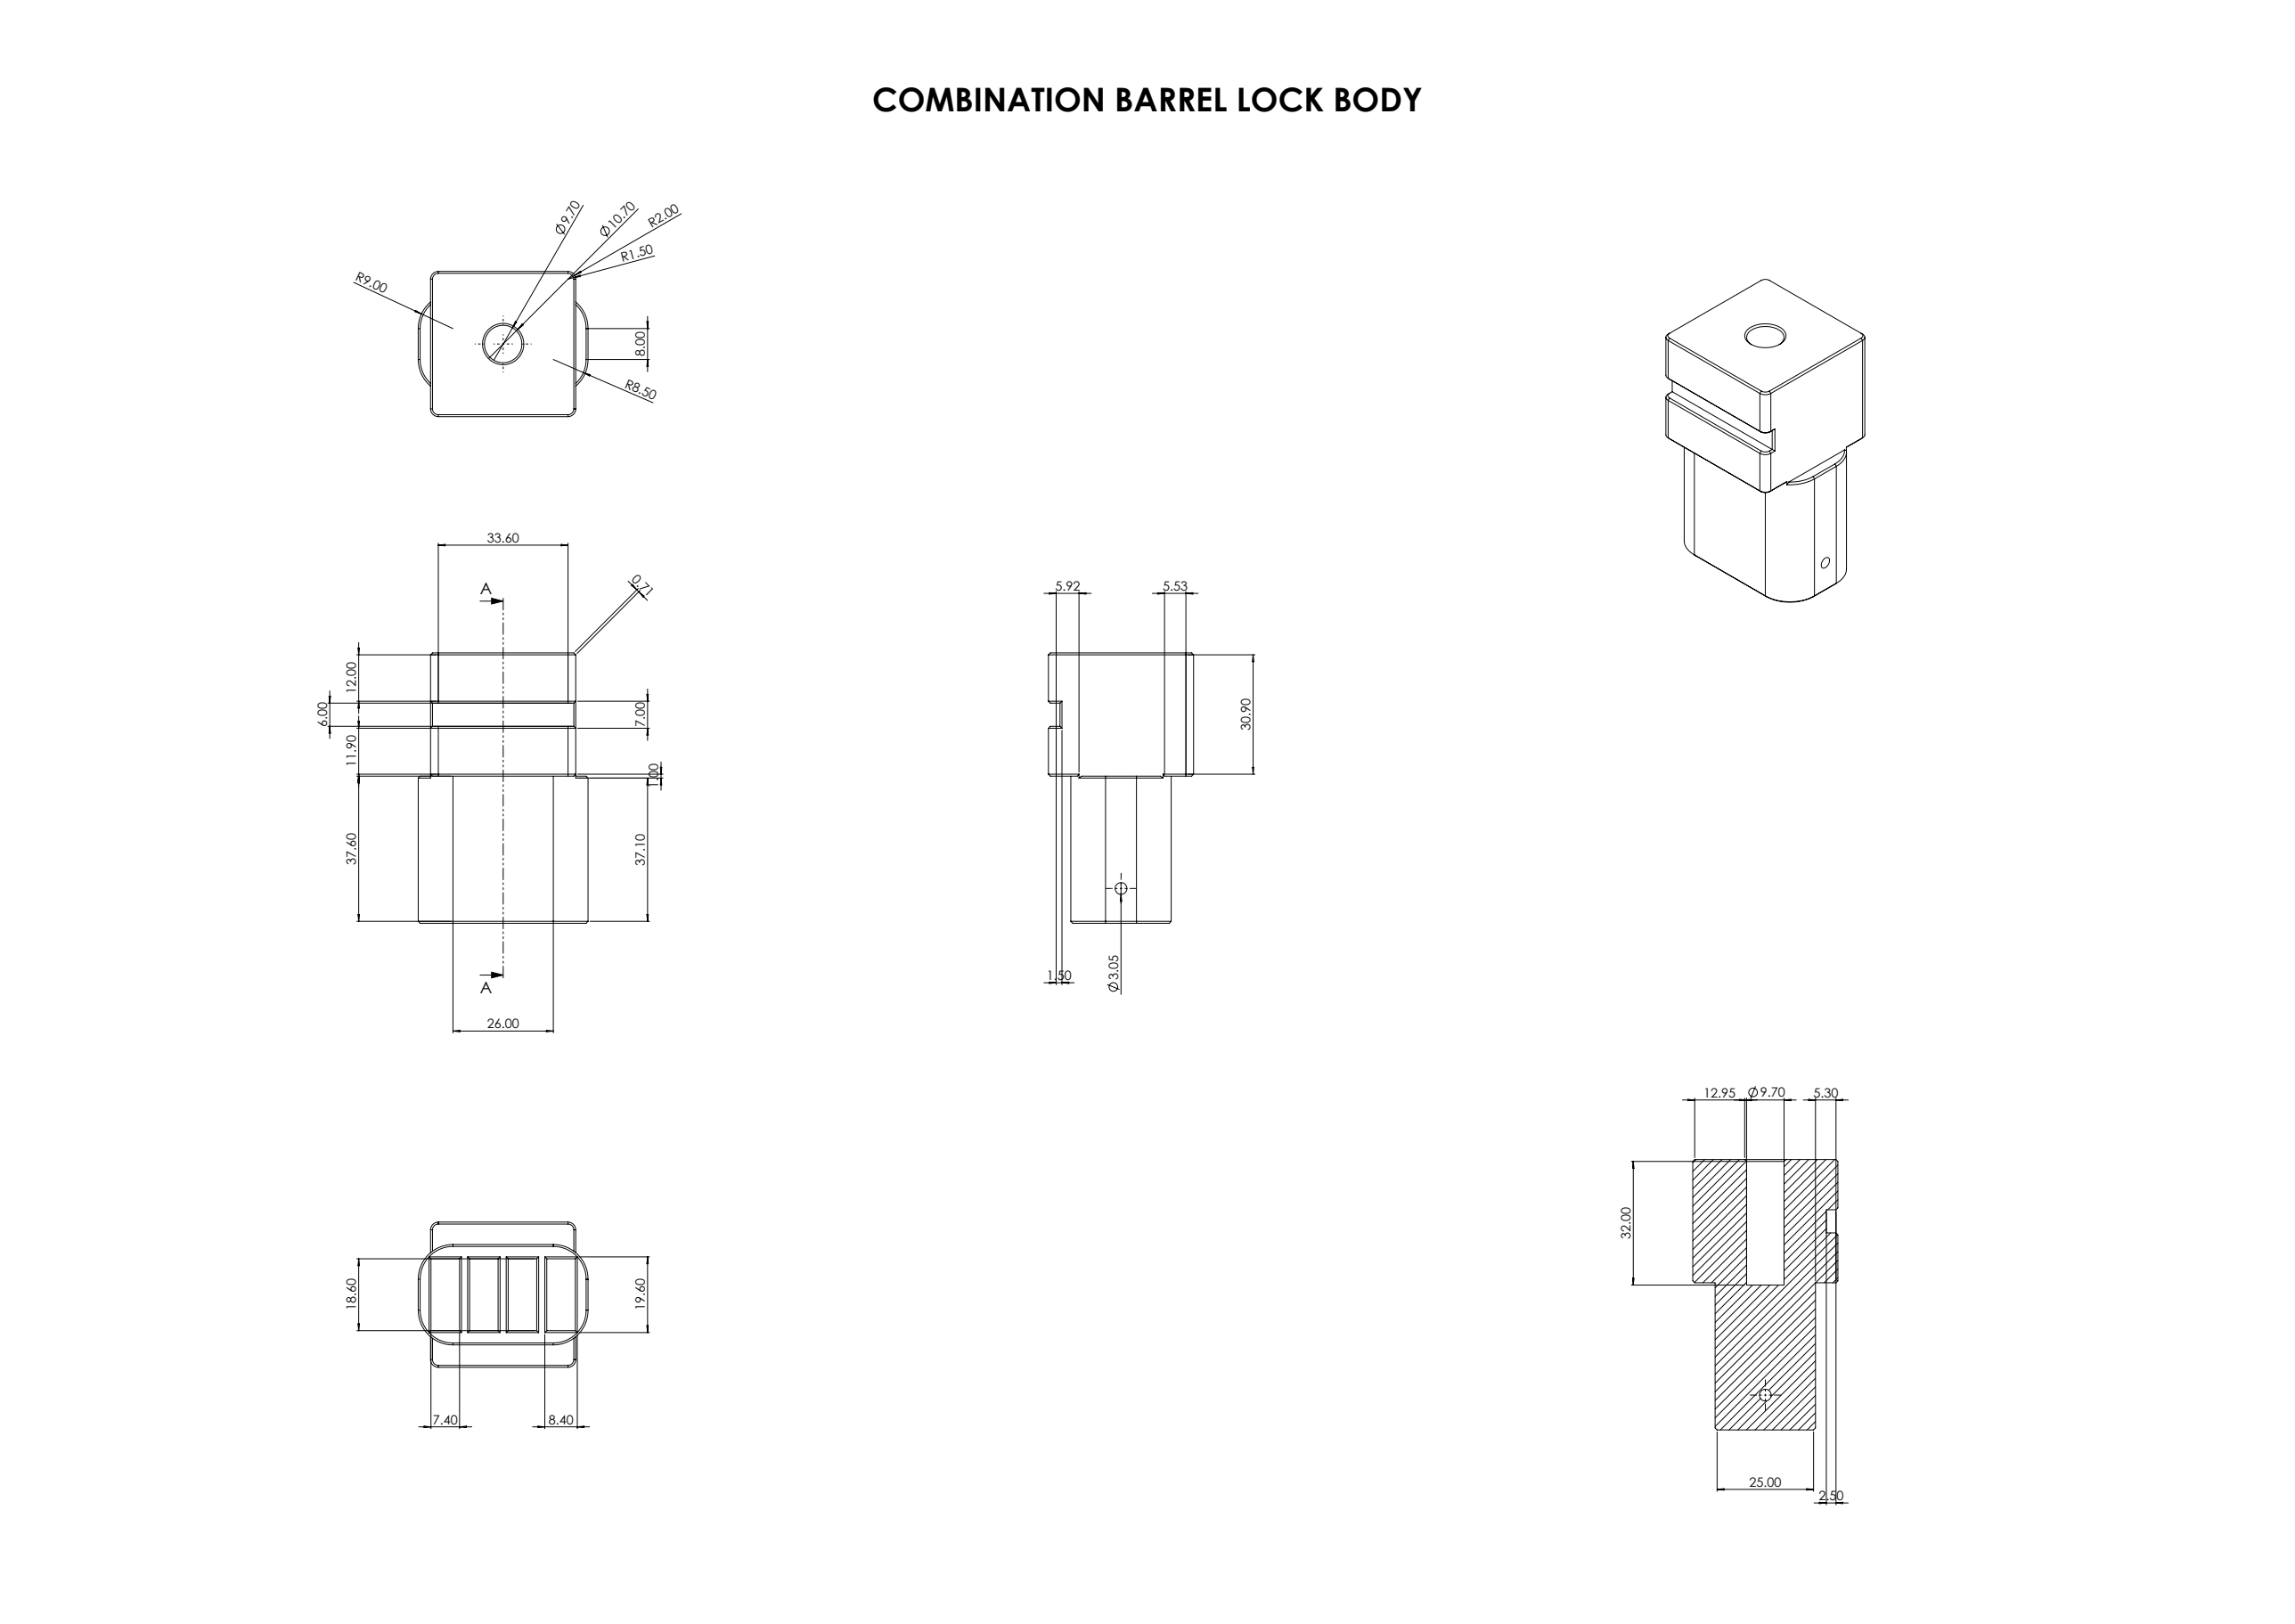
ISO-10303-21;
HEADER;
/* Generated by software containing ST-Developer
 * from STEP Tools, Inc. (www.steptools.com) 
 */

FILE_DESCRIPTION(
/* description */ (''),
/* implementation_level */ '2;1');

FILE_NAME(
/* name */ '08_Combination_Barrel_Lock_Body.step',
/* time_stamp */ '2026-10-25T01:30:15-07:00',
/* author */ (''),
/* organization */ (''),
/* preprocessor_version */ 'ST-DEVELOPER v20.2',
/* originating_system */ 'Autodesk Translation Framework v15.15.0.0',
/* authorisation */ '');

FILE_SCHEMA (('AUTOMOTIVE_DESIGN { 1 0 10303 214 3 1 1 }'));
ENDSEC;

DATA;
#10=MECHANICAL_DESIGN_GEOMETRIC_PRESENTATION_REPRESENTATION('',(#570),#32309);
#79=ELLIPSE('',#14443,12.7279220613578,8.99999999999999);
#80=ELLIPSE('',#14447,12.7279220613579,9.);
#81=ELLIPSE('',#14470,12.7279220613578,9.);
#82=ELLIPSE('',#14474,12.7279220613578,9.);
#83=(
BOUNDED_CURVE()
B_SPLINE_CURVE(2,(#25941,#25942,#25943),.UNSPECIFIED.,.F.,.F.)
B_SPLINE_CURVE_WITH_KNOTS((3,3),(0.,0.083454512499127),.UNSPECIFIED.)
CURVE()
GEOMETRIC_REPRESENTATION_ITEM()
RATIONAL_B_SPLINE_CURVE((1.,1.00072968826169,1.))
REPRESENTATION_ITEM('')
);
#84=(
BOUNDED_CURVE()
B_SPLINE_CURVE(2,(#25958,#25959,#25960),.UNSPECIFIED.,.F.,.F.)
B_SPLINE_CURVE_WITH_KNOTS((3,3),(0.,0.0834545124991277),.UNSPECIFIED.)
CURVE()
GEOMETRIC_REPRESENTATION_ITEM()
RATIONAL_B_SPLINE_CURVE((1.,1.00072968826163,1.))
REPRESENTATION_ITEM('')
);
#85=(
BOUNDED_CURVE()
B_SPLINE_CURVE(2,(#26021,#26022,#26023),.UNSPECIFIED.,.F.,.F.)
B_SPLINE_CURVE_WITH_KNOTS((3,3),(0.,0.0834545124991279),.UNSPECIFIED.)
CURVE()
GEOMETRIC_REPRESENTATION_ITEM()
RATIONAL_B_SPLINE_CURVE((1.,1.00072968826024,1.))
REPRESENTATION_ITEM('')
);
#86=(
BOUNDED_CURVE()
B_SPLINE_CURVE(2,(#26038,#26039,#26040),.UNSPECIFIED.,.F.,.F.)
B_SPLINE_CURVE_WITH_KNOTS((3,3),(0.,0.083454512499128),.UNSPECIFIED.)
CURVE()
GEOMETRIC_REPRESENTATION_ITEM()
RATIONAL_B_SPLINE_CURVE((1.,1.0007296882565,1.))
REPRESENTATION_ITEM('')
);
#542=SHAPE_REPRESENTATION_RELATIONSHIP('SRR','None',#32369,#556);
#556=ADVANCED_BREP_SHAPE_REPRESENTATION('',(#584),#32302);
#570=STYLED_ITEM('',(#32481),#584);
#584=MANIFOLD_SOLID_BREP('Body1',#13811);
#627=FACE_BOUND('',#2435,.T.);
#628=FACE_BOUND('',#2439,.T.);
#629=FACE_BOUND('',#2446,.T.);
#630=FACE_BOUND('',#2488,.T.);
#631=FACE_BOUND('',#2489,.T.);
#632=FACE_BOUND('',#2490,.T.);
#633=FACE_BOUND('',#2491,.T.);
#634=FACE_BOUND('',#2510,.T.);
#635=FACE_BOUND('',#2517,.T.);
#636=FACE_BOUND('',#2524,.T.);
#637=FACE_BOUND('',#2531,.T.);
#638=FACE_BOUND('',#2539,.T.);
#639=FACE_BOUND('',#2543,.T.);
#640=FACE_BOUND('',#2547,.T.);
#641=FACE_BOUND('',#2551,.T.);
#726=CYLINDRICAL_SURFACE('',#14440,8.99999999999999);
#727=CYLINDRICAL_SURFACE('',#14446,9.);
#728=CYLINDRICAL_SURFACE('',#14458,4.85);
#729=CYLINDRICAL_SURFACE('',#14467,9.);
#730=CYLINDRICAL_SURFACE('',#14473,9.);
#731=CYLINDRICAL_SURFACE('',#14487,2.);
#732=CYLINDRICAL_SURFACE('',#14490,2.);
#733=CYLINDRICAL_SURFACE('',#14502,2.);
#734=CYLINDRICAL_SURFACE('',#14505,2.);
#735=CYLINDRICAL_SURFACE('',#14517,2.);
#736=CYLINDRICAL_SURFACE('',#14581,1.525);
#737=CYLINDRICAL_SURFACE('',#14583,1.525);
#738=CYLINDRICAL_SURFACE('',#14585,1.525);
#739=CYLINDRICAL_SURFACE('',#14587,1.525);
#740=CYLINDRICAL_SURFACE('',#14589,1.525);
#741=CYLINDRICAL_SURFACE('',#14603,2.);
#951=CIRCLE('',#14434,9.);
#952=CIRCLE('',#14435,8.5);
#953=CIRCLE('',#14438,8.49999999999999);
#954=CIRCLE('',#14439,8.99999999999999);
#955=CIRCLE('',#14441,8.99999999999999);
#956=CIRCLE('',#14442,8.99999999999999);
#957=CIRCLE('',#14445,1.525);
#958=CIRCLE('',#14448,9.);
#959=CIRCLE('',#14449,9.);
#960=CIRCLE('',#14451,5.35);
#961=CIRCLE('',#14452,4.85);
#962=CIRCLE('',#14454,1.5);
#963=CIRCLE('',#14455,1.5);
#964=CIRCLE('',#14456,1.5);
#965=CIRCLE('',#14457,1.5);
#966=CIRCLE('',#14459,4.85);
#967=CIRCLE('',#14461,9.);
#968=CIRCLE('',#14462,8.5);
#969=CIRCLE('',#14465,8.5);
#970=CIRCLE('',#14466,9.);
#971=CIRCLE('',#14468,9.);
#972=CIRCLE('',#14469,9.);
#973=CIRCLE('',#14472,1.525);
#974=CIRCLE('',#14475,9.);
#975=CIRCLE('',#14476,9.);
#976=CIRCLE('',#14479,1.5);
#977=CIRCLE('',#14480,2.);
#978=CIRCLE('',#14483,1.5);
#979=CIRCLE('',#14484,2.);
#980=CIRCLE('',#14488,2.);
#981=CIRCLE('',#14491,2.);
#982=CIRCLE('',#14495,1.5);
#983=CIRCLE('',#14496,2.);
#984=CIRCLE('',#14499,1.5);
#985=CIRCLE('',#14500,2.);
#986=CIRCLE('',#14503,2.);
#987=CIRCLE('',#14506,2.);
#988=CIRCLE('',#14508,2.);
#989=CIRCLE('',#14515,2.);
#990=CIRCLE('',#14518,2.);
#991=CIRCLE('',#14523,8.49999999999999);
#992=CIRCLE('',#14526,8.5);
#993=CIRCLE('',#14529,8.5);
#994=CIRCLE('',#14532,8.5);
#995=CIRCLE('',#14538,2.);
#996=CIRCLE('',#14539,1.5);
#997=CIRCLE('',#14542,1.5);
#998=CIRCLE('',#14547,1.5);
#999=CIRCLE('',#14550,1.5);
#1000=CIRCLE('',#14559,1.525);
#1001=CIRCLE('',#14566,1.525);
#1002=CIRCLE('',#14573,1.525);
#1003=CIRCLE('',#14580,1.525);
#1004=CIRCLE('',#14582,1.525);
#1005=CIRCLE('',#14584,1.525);
#1006=CIRCLE('',#14586,1.525);
#1007=CIRCLE('',#14588,1.525);
#1181=CONICAL_SURFACE('',#14433,8.75,0.785398163397444);
#1182=CONICAL_SURFACE('',#14437,8.75,0.785398163397449);
#1183=CONICAL_SURFACE('',#14450,5.1,0.785398163397447);
#1184=CONICAL_SURFACE('',#14460,8.75,0.785398163397449);
#1185=CONICAL_SURFACE('',#14464,8.75,0.785398163397451);
#1186=CONICAL_SURFACE('',#14478,1.75,0.785398163397449);
#1187=CONICAL_SURFACE('',#14482,1.75,0.785398163397449);
#1188=CONICAL_SURFACE('',#14494,1.75,0.785398163397449);
#1189=CONICAL_SURFACE('',#14498,1.75,0.785398163397449);
#1190=CONICAL_SURFACE('',#14507,1.75,0.785398163397447);
#1191=CONICAL_SURFACE('',#14510,1.75,0.785398163397447);
#1192=CONICAL_SURFACE('',#14512,1.75,0.785398163397447);
#1193=CONICAL_SURFACE('',#14514,1.75,0.785398163397447);
#1194=CONICAL_SURFACE('',#14522,8.75,0.785398163397449);
#1195=CONICAL_SURFACE('',#14525,8.75,0.785398163397449);
#1196=CONICAL_SURFACE('',#14528,8.75,0.785398163397449);
#1197=CONICAL_SURFACE('',#14531,8.75,0.785398163397449);
#1198=CONICAL_SURFACE('',#14537,1.75,0.785398163397447);
#1199=CONICAL_SURFACE('',#14541,1.75,0.785398163397447);
#1200=CONICAL_SURFACE('',#14546,1.75,0.785398163397447);
#1201=CONICAL_SURFACE('',#14549,1.75,0.785398163397447);
#1595=FACE_OUTER_BOUND('',#2430,.T.);
#1596=FACE_OUTER_BOUND('',#2431,.T.);
#1597=FACE_OUTER_BOUND('',#2432,.T.);
#1598=FACE_OUTER_BOUND('',#2433,.T.);
#1599=FACE_OUTER_BOUND('',#2434,.T.);
#1600=FACE_OUTER_BOUND('',#2436,.T.);
#1601=FACE_OUTER_BOUND('',#2437,.T.);
#1602=FACE_OUTER_BOUND('',#2438,.T.);
#1603=FACE_OUTER_BOUND('',#2440,.T.);
#1604=FACE_OUTER_BOUND('',#2441,.T.);
#1605=FACE_OUTER_BOUND('',#2442,.T.);
#1606=FACE_OUTER_BOUND('',#2443,.T.);
#1607=FACE_OUTER_BOUND('',#2444,.T.);
#1608=FACE_OUTER_BOUND('',#2445,.T.);
#1609=FACE_OUTER_BOUND('',#2447,.T.);
#1610=FACE_OUTER_BOUND('',#2448,.T.);
#1611=FACE_OUTER_BOUND('',#2449,.T.);
#1612=FACE_OUTER_BOUND('',#2450,.T.);
#1613=FACE_OUTER_BOUND('',#2451,.T.);
#1614=FACE_OUTER_BOUND('',#2452,.T.);
#1615=FACE_OUTER_BOUND('',#2453,.T.);
#1616=FACE_OUTER_BOUND('',#2454,.T.);
#1617=FACE_OUTER_BOUND('',#2455,.T.);
#1618=FACE_OUTER_BOUND('',#2456,.T.);
#1619=FACE_OUTER_BOUND('',#2457,.T.);
#1620=FACE_OUTER_BOUND('',#2458,.T.);
#1621=FACE_OUTER_BOUND('',#2459,.T.);
#1622=FACE_OUTER_BOUND('',#2460,.T.);
#1623=FACE_OUTER_BOUND('',#2461,.T.);
#1624=FACE_OUTER_BOUND('',#2462,.T.);
#1625=FACE_OUTER_BOUND('',#2463,.T.);
#1626=FACE_OUTER_BOUND('',#2464,.T.);
#1627=FACE_OUTER_BOUND('',#2465,.T.);
#1628=FACE_OUTER_BOUND('',#2466,.T.);
#1629=FACE_OUTER_BOUND('',#2467,.T.);
#1630=FACE_OUTER_BOUND('',#2468,.T.);
#1631=FACE_OUTER_BOUND('',#2469,.T.);
#1632=FACE_OUTER_BOUND('',#2470,.T.);
#1633=FACE_OUTER_BOUND('',#2471,.T.);
#1634=FACE_OUTER_BOUND('',#2472,.T.);
#1635=FACE_OUTER_BOUND('',#2473,.T.);
#1636=FACE_OUTER_BOUND('',#2474,.T.);
#1637=FACE_OUTER_BOUND('',#2475,.T.);
#1638=FACE_OUTER_BOUND('',#2476,.T.);
#1639=FACE_OUTER_BOUND('',#2477,.T.);
#1640=FACE_OUTER_BOUND('',#2478,.T.);
#1641=FACE_OUTER_BOUND('',#2479,.T.);
#1642=FACE_OUTER_BOUND('',#2480,.T.);
#1643=FACE_OUTER_BOUND('',#2481,.T.);
#1644=FACE_OUTER_BOUND('',#2482,.T.);
#1645=FACE_OUTER_BOUND('',#2483,.T.);
#1646=FACE_OUTER_BOUND('',#2484,.T.);
#1647=FACE_OUTER_BOUND('',#2485,.T.);
#1648=FACE_OUTER_BOUND('',#2486,.T.);
#1649=FACE_OUTER_BOUND('',#2487,.T.);
#1650=FACE_OUTER_BOUND('',#2492,.T.);
#1651=FACE_OUTER_BOUND('',#2493,.T.);
#1652=FACE_OUTER_BOUND('',#2494,.T.);
#1653=FACE_OUTER_BOUND('',#2495,.T.);
#1654=FACE_OUTER_BOUND('',#2496,.T.);
#1655=FACE_OUTER_BOUND('',#2497,.T.);
#1656=FACE_OUTER_BOUND('',#2498,.T.);
#1657=FACE_OUTER_BOUND('',#2499,.T.);
#1658=FACE_OUTER_BOUND('',#2500,.T.);
#1659=FACE_OUTER_BOUND('',#2501,.T.);
#1660=FACE_OUTER_BOUND('',#2502,.T.);
#1661=FACE_OUTER_BOUND('',#2503,.T.);
#1662=FACE_OUTER_BOUND('',#2504,.T.);
#1663=FACE_OUTER_BOUND('',#2505,.T.);
#1664=FACE_OUTER_BOUND('',#2506,.T.);
#1665=FACE_OUTER_BOUND('',#2507,.T.);
#1666=FACE_OUTER_BOUND('',#2508,.T.);
#1667=FACE_OUTER_BOUND('',#2509,.T.);
#1668=FACE_OUTER_BOUND('',#2511,.T.);
#1669=FACE_OUTER_BOUND('',#2512,.T.);
#1670=FACE_OUTER_BOUND('',#2513,.T.);
#1671=FACE_OUTER_BOUND('',#2514,.T.);
#1672=FACE_OUTER_BOUND('',#2515,.T.);
#1673=FACE_OUTER_BOUND('',#2516,.T.);
#1674=FACE_OUTER_BOUND('',#2518,.T.);
#1675=FACE_OUTER_BOUND('',#2519,.T.);
#1676=FACE_OUTER_BOUND('',#2520,.T.);
#1677=FACE_OUTER_BOUND('',#2521,.T.);
#1678=FACE_OUTER_BOUND('',#2522,.T.);
#1679=FACE_OUTER_BOUND('',#2523,.T.);
#1680=FACE_OUTER_BOUND('',#2525,.T.);
#1681=FACE_OUTER_BOUND('',#2526,.T.);
#1682=FACE_OUTER_BOUND('',#2527,.T.);
#1683=FACE_OUTER_BOUND('',#2528,.T.);
#1684=FACE_OUTER_BOUND('',#2529,.T.);
#1685=FACE_OUTER_BOUND('',#2530,.T.);
#1686=FACE_OUTER_BOUND('',#2532,.T.);
#1687=FACE_OUTER_BOUND('',#2533,.T.);
#1688=FACE_OUTER_BOUND('',#2534,.T.);
#1689=FACE_OUTER_BOUND('',#2535,.T.);
#1690=FACE_OUTER_BOUND('',#2536,.T.);
#1691=FACE_OUTER_BOUND('',#2537,.T.);
#1692=FACE_OUTER_BOUND('',#2538,.T.);
#1693=FACE_OUTER_BOUND('',#2540,.T.);
#1694=FACE_OUTER_BOUND('',#2541,.T.);
#1695=FACE_OUTER_BOUND('',#2542,.T.);
#1696=FACE_OUTER_BOUND('',#2544,.T.);
#1697=FACE_OUTER_BOUND('',#2545,.T.);
#1698=FACE_OUTER_BOUND('',#2546,.T.);
#1699=FACE_OUTER_BOUND('',#2548,.T.);
#1700=FACE_OUTER_BOUND('',#2549,.T.);
#1701=FACE_OUTER_BOUND('',#2550,.T.);
#1702=FACE_OUTER_BOUND('',#2552,.T.);
#1703=FACE_OUTER_BOUND('',#2553,.T.);
#1704=FACE_OUTER_BOUND('',#2554,.T.);
#1705=FACE_OUTER_BOUND('',#2555,.T.);
#1706=FACE_OUTER_BOUND('',#2556,.T.);
#1707=FACE_OUTER_BOUND('',#2557,.T.);
#1708=FACE_OUTER_BOUND('',#2558,.T.);
#1709=FACE_OUTER_BOUND('',#2559,.T.);
#1710=FACE_OUTER_BOUND('',#2560,.T.);
#2430=EDGE_LOOP('',(#10369,#10370,#10371,#10372));
#2431=EDGE_LOOP('',(#10373,#10374,#10375,#10376));
#2432=EDGE_LOOP('',(#10377,#10378,#10379,#10380));
#2433=EDGE_LOOP('',(#10381,#10382,#10383,#10384,#10385,#10386,#10387));
#2434=EDGE_LOOP('',(#10388,#10389,#10390,#10391));
#2435=EDGE_LOOP('',(#10392));
#2436=EDGE_LOOP('',(#10393,#10394,#10395,#10396,#10397,#10398,#10399));
#2437=EDGE_LOOP('',(#10400,#10401,#10402,#10403));
#2438=EDGE_LOOP('',(#10404,#10405,#10406,#10407,#10408,#10409,#10410,#10411));
#2439=EDGE_LOOP('',(#10412));
#2440=EDGE_LOOP('',(#10413,#10414,#10415,#10416));
#2441=EDGE_LOOP('',(#10417,#10418,#10419,#10420));
#2442=EDGE_LOOP('',(#10421,#10422,#10423,#10424));
#2443=EDGE_LOOP('',(#10425,#10426,#10427,#10428));
#2444=EDGE_LOOP('',(#10429,#10430,#10431,#10432,#10433,#10434,#10435));
#2445=EDGE_LOOP('',(#10436,#10437,#10438,#10439));
#2446=EDGE_LOOP('',(#10440));
#2447=EDGE_LOOP('',(#10441,#10442,#10443,#10444,#10445,#10446,#10447));
#2448=EDGE_LOOP('',(#10448,#10449,#10450,#10451));
#2449=EDGE_LOOP('',(#10452,#10453,#10454,#10455));
#2450=EDGE_LOOP('',(#10456,#10457,#10458,#10459));
#2451=EDGE_LOOP('',(#10460,#10461,#10462,#10463));
#2452=EDGE_LOOP('',(#10464,#10465,#10466,#10467));
#2453=EDGE_LOOP('',(#10468,#10469,#10470,#10471,#10472,#10473,#10474,#10475,
#10476,#10477,#10478,#10479,#10480,#10481));
#2454=EDGE_LOOP('',(#10482,#10483,#10484,#10485));
#2455=EDGE_LOOP('',(#10486,#10487,#10488,#10489));
#2456=EDGE_LOOP('',(#10490,#10491,#10492,#10493));
#2457=EDGE_LOOP('',(#10494,#10495,#10496,#10497,#10498,#10499,#10500,#10501,
#10502,#10503,#10504,#10505,#10506,#10507));
#2458=EDGE_LOOP('',(#10508,#10509,#10510,#10511));
#2459=EDGE_LOOP('',(#10512,#10513,#10514,#10515));
#2460=EDGE_LOOP('',(#10516,#10517,#10518,#10519));
#2461=EDGE_LOOP('',(#10520,#10521,#10522,#10523));
#2462=EDGE_LOOP('',(#10524,#10525,#10526,#10527));
#2463=EDGE_LOOP('',(#10528,#10529,#10530,#10531));
#2464=EDGE_LOOP('',(#10532,#10533,#10534,#10535));
#2465=EDGE_LOOP('',(#10536,#10537,#10538,#10539));
#2466=EDGE_LOOP('',(#10540,#10541,#10542,#10543));
#2467=EDGE_LOOP('',(#10544,#10545,#10546,#10547));
#2468=EDGE_LOOP('',(#10548,#10549,#10550,#10551));
#2469=EDGE_LOOP('',(#10552,#10553,#10554,#10555));
#2470=EDGE_LOOP('',(#10556,#10557,#10558,#10559));
#2471=EDGE_LOOP('',(#10560,#10561,#10562,#10563));
#2472=EDGE_LOOP('',(#10564,#10565,#10566,#10567));
#2473=EDGE_LOOP('',(#10568,#10569,#10570,#10571));
#2474=EDGE_LOOP('',(#10572,#10573,#10574,#10575));
#2475=EDGE_LOOP('',(#10576,#10577,#10578,#10579));
#2476=EDGE_LOOP('',(#10580,#10581,#10582,#10583));
#2477=EDGE_LOOP('',(#10584,#10585,#10586,#10587));
#2478=EDGE_LOOP('',(#10588,#10589,#10590,#10591));
#2479=EDGE_LOOP('',(#10592,#10593,#10594,#10595));
#2480=EDGE_LOOP('',(#10596,#10597,#10598,#10599));
#2481=EDGE_LOOP('',(#10600,#10601,#10602,#10603));
#2482=EDGE_LOOP('',(#10604,#10605,#10606,#10607));
#2483=EDGE_LOOP('',(#10608,#10609,#10610,#10611));
#2484=EDGE_LOOP('',(#10612,#10613,#10614,#10615));
#2485=EDGE_LOOP('',(#10616,#10617,#10618,#10619));
#2486=EDGE_LOOP('',(#10620,#10621,#10622,#10623));
#2487=EDGE_LOOP('',(#10624,#10625,#10626,#10627,#10628,#10629,#10630,#10631));
#2488=EDGE_LOOP('',(#10632,#10633,#10634,#10635));
#2489=EDGE_LOOP('',(#10636,#10637,#10638,#10639));
#2490=EDGE_LOOP('',(#10640,#10641,#10642,#10643));
#2491=EDGE_LOOP('',(#10644,#10645,#10646,#10647));
#2492=EDGE_LOOP('',(#10648,#10649,#10650,#10651));
#2493=EDGE_LOOP('',(#10652,#10653,#10654,#10655));
#2494=EDGE_LOOP('',(#10656,#10657,#10658,#10659));
#2495=EDGE_LOOP('',(#10660,#10661,#10662,#10663));
#2496=EDGE_LOOP('',(#10664,#10665,#10666,#10667));
#2497=EDGE_LOOP('',(#10668,#10669,#10670,#10671,#10672,#10673));
#2498=EDGE_LOOP('',(#10674,#10675,#10676,#10677));
#2499=EDGE_LOOP('',(#10678,#10679,#10680,#10681));
#2500=EDGE_LOOP('',(#10682,#10683,#10684,#10685));
#2501=EDGE_LOOP('',(#10686,#10687,#10688,#10689));
#2502=EDGE_LOOP('',(#10690,#10691,#10692,#10693));
#2503=EDGE_LOOP('',(#10694,#10695,#10696,#10697,#10698,#10699));
#2504=EDGE_LOOP('',(#10700,#10701,#10702,#10703));
#2505=EDGE_LOOP('',(#10704,#10705,#10706,#10707));
#2506=EDGE_LOOP('',(#10708,#10709,#10710,#10711));
#2507=EDGE_LOOP('',(#10712,#10713,#10714,#10715));
#2508=EDGE_LOOP('',(#10716,#10717,#10718,#10719));
#2509=EDGE_LOOP('',(#10720,#10721,#10722,#10723));
#2510=EDGE_LOOP('',(#10724));
#2511=EDGE_LOOP('',(#10725,#10726,#10727,#10728));
#2512=EDGE_LOOP('',(#10729,#10730,#10731,#10732));
#2513=EDGE_LOOP('',(#10733,#10734,#10735,#10736));
#2514=EDGE_LOOP('',(#10737,#10738,#10739,#10740));
#2515=EDGE_LOOP('',(#10741,#10742,#10743,#10744));
#2516=EDGE_LOOP('',(#10745,#10746,#10747,#10748));
#2517=EDGE_LOOP('',(#10749));
#2518=EDGE_LOOP('',(#10750,#10751,#10752,#10753));
#2519=EDGE_LOOP('',(#10754,#10755,#10756,#10757));
#2520=EDGE_LOOP('',(#10758,#10759,#10760,#10761));
#2521=EDGE_LOOP('',(#10762,#10763,#10764,#10765));
#2522=EDGE_LOOP('',(#10766,#10767,#10768,#10769));
#2523=EDGE_LOOP('',(#10770,#10771,#10772,#10773));
#2524=EDGE_LOOP('',(#10774));
#2525=EDGE_LOOP('',(#10775,#10776,#10777,#10778));
#2526=EDGE_LOOP('',(#10779,#10780,#10781,#10782));
#2527=EDGE_LOOP('',(#10783,#10784,#10785,#10786));
#2528=EDGE_LOOP('',(#10787,#10788,#10789,#10790));
#2529=EDGE_LOOP('',(#10791,#10792,#10793,#10794));
#2530=EDGE_LOOP('',(#10795,#10796,#10797,#10798));
#2531=EDGE_LOOP('',(#10799));
#2532=EDGE_LOOP('',(#10800,#10801,#10802,#10803));
#2533=EDGE_LOOP('',(#10804,#10805,#10806,#10807));
#2534=EDGE_LOOP('',(#10808,#10809,#10810,#10811));
#2535=EDGE_LOOP('',(#10812,#10813,#10814,#10815));
#2536=EDGE_LOOP('',(#10816,#10817,#10818,#10819));
#2537=EDGE_LOOP('',(#10820,#10821,#10822,#10823));
#2538=EDGE_LOOP('',(#10824,#10825,#10826,#10827));
#2539=EDGE_LOOP('',(#10828));
#2540=EDGE_LOOP('',(#10829,#10830,#10831,#10832));
#2541=EDGE_LOOP('',(#10833,#10834,#10835,#10836));
#2542=EDGE_LOOP('',(#10837,#10838,#10839,#10840));
#2543=EDGE_LOOP('',(#10841));
#2544=EDGE_LOOP('',(#10842,#10843,#10844,#10845));
#2545=EDGE_LOOP('',(#10846,#10847,#10848,#10849));
#2546=EDGE_LOOP('',(#10850,#10851,#10852,#10853));
#2547=EDGE_LOOP('',(#10854));
#2548=EDGE_LOOP('',(#10855,#10856,#10857,#10858));
#2549=EDGE_LOOP('',(#10859,#10860,#10861,#10862));
#2550=EDGE_LOOP('',(#10863,#10864,#10865,#10866));
#2551=EDGE_LOOP('',(#10867));
#2552=EDGE_LOOP('',(#10868,#10869,#10870,#10871));
#2553=EDGE_LOOP('',(#10872,#10873,#10874,#10875));
#2554=EDGE_LOOP('',(#10876,#10877,#10878,#10879));
#2555=EDGE_LOOP('',(#10880));
#2556=EDGE_LOOP('',(#10881,#10882,#10883,#10884));
#2557=EDGE_LOOP('',(#10885,#10886,#10887,#10888));
#2558=EDGE_LOOP('',(#10889,#10890,#10891,#10892));
#2559=EDGE_LOOP('',(#10893,#10894,#10895,#10896,#10897,#10898,#10899,#10900));
#2560=EDGE_LOOP('',(#10901,#10902,#10903,#10904,#10905,#10906,#10907,#10908));
#3355=LINE('',#25947,#4666);
#3356=LINE('',#25951,#4667);
#3357=LINE('',#25953,#4668);
#3358=LINE('',#25954,#4669);
#3359=LINE('',#25965,#4670);
#3360=LINE('',#25967,#4671);
#3361=LINE('',#25971,#4672);
#3362=LINE('',#25977,#4673);
#3363=LINE('',#25978,#4674);
#3364=LINE('',#25983,#4675);
#3365=LINE('',#25989,#4676);
#3366=LINE('',#25995,#4677);
#3367=LINE('',#26002,#4678);
#3368=LINE('',#26006,#4679);
#3369=LINE('',#26010,#4680);
#3370=LINE('',#26013,#4681);
#3371=LINE('',#26016,#4682);
#3372=LINE('',#26027,#4683);
#3373=LINE('',#26031,#4684);
#3374=LINE('',#26033,#4685);
#3375=LINE('',#26034,#4686);
#3376=LINE('',#26045,#4687);
#3377=LINE('',#26047,#4688);
#3378=LINE('',#26051,#4689);
#3379=LINE('',#26057,#4690);
#3380=LINE('',#26058,#4691);
#3381=LINE('',#26063,#4692);
#3382=LINE('',#26069,#4693);
#3383=LINE('',#26073,#4694);
#3384=LINE('',#26075,#4695);
#3385=LINE('',#26076,#4696);
#3386=LINE('',#26080,#4697);
#3387=LINE('',#26086,#4698);
#3388=LINE('',#26087,#4699);
#3389=LINE('',#26088,#4700);
#3390=LINE('',#26092,#4701);
#3391=LINE('',#26096,#4702);
#3392=LINE('',#26097,#4703);
#3393=LINE('',#26100,#4704);
#3394=LINE('',#26102,#4705);
#3395=LINE('',#26104,#4706);
#3396=LINE('',#26106,#4707);
#3397=LINE('',#26108,#4708);
#3398=LINE('',#26110,#4709);
#3399=LINE('',#26112,#4710);
#3400=LINE('',#26113,#4711);
#3401=LINE('',#26114,#4712);
#3402=LINE('',#26117,#4713);
#3403=LINE('',#26121,#4714);
#3404=LINE('',#26122,#4715);
#3405=LINE('',#26125,#4716);
#3406=LINE('',#26128,#4717);
#3407=LINE('',#26130,#4718);
#3408=LINE('',#26132,#4719);
#3409=LINE('',#26134,#4720);
#3410=LINE('',#26136,#4721);
#3411=LINE('',#26138,#4722);
#3412=LINE('',#26140,#4723);
#3413=LINE('',#26141,#4724);
#3414=LINE('',#26144,#4725);
#3415=LINE('',#26145,#4726);
#3416=LINE('',#26149,#4727);
#3417=LINE('',#26155,#4728);
#3418=LINE('',#26156,#4729);
#3419=LINE('',#26157,#4730);
#3420=LINE('',#26160,#4731);
#3421=LINE('',#26164,#4732);
#3422=LINE('',#26167,#4733);
#3423=LINE('',#26171,#4734);
#3424=LINE('',#26172,#4735);
#3425=LINE('',#26176,#4736);
#3426=LINE('',#26178,#4737);
#3427=LINE('',#26181,#4738);
#3428=LINE('',#26183,#4739);
#3429=LINE('',#26185,#4740);
#3430=LINE('',#26187,#4741);
#3431=LINE('',#26189,#4742);
#3432=LINE('',#26192,#4743);
#3433=LINE('',#26195,#4744);
#3434=LINE('',#26198,#4745);
#3435=LINE('',#26202,#4746);
#3436=LINE('',#26204,#4747);
#3437=LINE('',#26205,#4748);
#3438=LINE('',#26208,#4749);
#3439=LINE('',#26210,#4750);
#3440=LINE('',#26211,#4751);
#3441=LINE('',#26213,#4752);
#3442=LINE('',#26214,#4753);
#3443=LINE('',#26217,#4754);
#3444=LINE('',#26220,#4755);
#3445=LINE('',#26223,#4756);
#3446=LINE('',#26224,#4757);
#3447=LINE('',#26227,#4758);
#3448=LINE('',#26231,#4759);
#3449=LINE('',#26232,#4760);
#3450=LINE('',#26233,#4761);
#3451=LINE('',#26236,#4762);
#3452=LINE('',#26240,#4763);
#3453=LINE('',#26241,#4764);
#3454=LINE('',#26244,#4765);
#3455=LINE('',#26247,#4766);
#3456=LINE('',#26248,#4767);
#3457=LINE('',#26250,#4768);
#3458=LINE('',#26254,#4769);
#3459=LINE('',#26256,#4770);
#3460=LINE('',#26258,#4771);
#3461=LINE('',#26259,#4772);
#3462=LINE('',#26262,#4773);
#3463=LINE('',#26264,#4774);
#3464=LINE('',#26266,#4775);
#3465=LINE('',#26267,#4776);
#3466=LINE('',#26270,#4777);
#3467=LINE('',#26272,#4778);
#3468=LINE('',#26274,#4779);
#3469=LINE('',#26275,#4780);
#3470=LINE('',#26278,#4781);
#3471=LINE('',#26280,#4782);
#3472=LINE('',#26282,#4783);
#3473=LINE('',#26283,#4784);
#3474=LINE('',#26286,#4785);
#3475=LINE('',#26287,#4786);
#3476=LINE('',#26291,#4787);
#3477=LINE('',#26296,#4788);
#3478=LINE('',#26297,#4789);
#3479=LINE('',#26298,#4790);
#3480=LINE('',#26301,#4791);
#3481=LINE('',#26304,#4792);
#3482=LINE('',#26308,#4793);
#3483=LINE('',#26309,#4794);
#3484=LINE('',#26312,#4795);
#3485=LINE('',#26316,#4796);
#3486=LINE('',#26317,#4797);
#3487=LINE('',#26320,#4798);
#3488=LINE('',#26323,#4799);
#3489=LINE('',#26327,#4800);
#3490=LINE('',#26329,#4801);
#3491=LINE('',#26330,#4802);
#3492=LINE('',#26333,#4803);
#3493=LINE('',#26335,#4804);
#3494=LINE('',#26336,#4805);
#3495=LINE('',#26338,#4806);
#3496=LINE('',#26340,#4807);
#3497=LINE('',#26343,#4808);
#3498=LINE('',#26345,#4809);
#3499=LINE('',#26346,#4810);
#3500=LINE('',#26349,#4811);
#3501=LINE('',#26350,#4812);
#3502=LINE('',#26355,#4813);
#3503=LINE('',#26357,#4814);
#3504=LINE('',#26358,#4815);
#3505=LINE('',#26361,#4816);
#3506=LINE('',#26363,#4817);
#3507=LINE('',#26364,#4818);
#3508=LINE('',#26366,#4819);
#3509=LINE('',#26368,#4820);
#3510=LINE('',#26371,#4821);
#3511=LINE('',#26373,#4822);
#3512=LINE('',#26374,#4823);
#3513=LINE('',#26377,#4824);
#3514=LINE('',#26378,#4825);
#3515=LINE('',#26383,#4826);
#3516=LINE('',#26385,#4827);
#3517=LINE('',#26386,#4828);
#3518=LINE('',#26389,#4829);
#3519=LINE('',#26391,#4830);
#3520=LINE('',#26392,#4831);
#3521=LINE('',#26394,#4832);
#3522=LINE('',#26396,#4833);
#3523=LINE('',#26399,#4834);
#3524=LINE('',#26401,#4835);
#3525=LINE('',#26402,#4836);
#3526=LINE('',#26405,#4837);
#3527=LINE('',#26406,#4838);
#3528=LINE('',#26411,#4839);
#3529=LINE('',#26413,#4840);
#3530=LINE('',#26414,#4841);
#3531=LINE('',#26417,#4842);
#3532=LINE('',#26419,#4843);
#3533=LINE('',#26420,#4844);
#3534=LINE('',#26422,#4845);
#3535=LINE('',#26424,#4846);
#3536=LINE('',#26427,#4847);
#3537=LINE('',#26429,#4848);
#3538=LINE('',#26430,#4849);
#3539=LINE('',#26433,#4850);
#3540=LINE('',#26434,#4851);
#3541=LINE('',#26439,#4852);
#3542=LINE('',#26443,#4853);
#3543=LINE('',#26447,#4854);
#3544=LINE('',#26451,#4855);
#3545=LINE('',#26454,#4856);
#3546=LINE('',#26457,#4857);
#3547=LINE('',#26458,#4858);
#3548=LINE('',#26460,#4859);
#3549=LINE('',#26464,#4860);
#3550=LINE('',#26465,#4861);
#3551=LINE('',#26467,#4862);
#3552=LINE('',#26471,#4863);
#3553=LINE('',#26472,#4864);
#3554=LINE('',#26474,#4865);
#3555=LINE('',#26478,#4866);
#3556=LINE('',#26479,#4867);
#3557=LINE('',#26481,#4868);
#3558=LINE('',#26484,#4869);
#3559=LINE('',#26490,#4870);
#4666=VECTOR('',#16387,10.);
#4667=VECTOR('',#16392,10.);
#4668=VECTOR('',#16393,10.);
#4669=VECTOR('',#16394,10.);
#4670=VECTOR('',#16403,10.);
#4671=VECTOR('',#16404,10.);
#4672=VECTOR('',#16407,10.);
#4673=VECTOR('',#16414,10.);
#4674=VECTOR('',#16415,10.);
#4675=VECTOR('',#16420,10.);
#4676=VECTOR('',#16425,10.);
#4677=VECTOR('',#16432,5.1);
#4678=VECTOR('',#16439,10.);
#4679=VECTOR('',#16442,10.);
#4680=VECTOR('',#16445,10.);
#4681=VECTOR('',#16448,10.);
#4682=VECTOR('',#16451,4.85);
#4683=VECTOR('',#16458,10.);
#4684=VECTOR('',#16463,10.);
#4685=VECTOR('',#16464,10.);
#4686=VECTOR('',#16465,10.);
#4687=VECTOR('',#16474,10.);
#4688=VECTOR('',#16475,10.);
#4689=VECTOR('',#16478,10.);
#4690=VECTOR('',#16485,10.);
#4691=VECTOR('',#16486,10.);
#4692=VECTOR('',#16491,10.);
#4693=VECTOR('',#16496,10.);
#4694=VECTOR('',#16501,10.);
#4695=VECTOR('',#16502,10.);
#4696=VECTOR('',#16503,10.);
#4697=VECTOR('',#16506,10.);
#4698=VECTOR('',#16513,10.);
#4699=VECTOR('',#16514,10.);
#4700=VECTOR('',#16515,10.);
#4701=VECTOR('',#16518,10.);
#4702=VECTOR('',#16525,10.);
#4703=VECTOR('',#16526,10.);
#4704=VECTOR('',#16529,10.);
#4705=VECTOR('',#16530,10.);
#4706=VECTOR('',#16531,10.);
#4707=VECTOR('',#16532,10.);
#4708=VECTOR('',#16533,10.);
#4709=VECTOR('',#16534,10.);
#4710=VECTOR('',#16535,10.);
#4711=VECTOR('',#16536,10.);
#4712=VECTOR('',#16537,10.);
#4713=VECTOR('',#16540,10.);
#4714=VECTOR('',#16545,10.);
#4715=VECTOR('',#16546,10.);
#4716=VECTOR('',#16549,10.);
#4717=VECTOR('',#16554,10.);
#4718=VECTOR('',#16555,10.);
#4719=VECTOR('',#16556,10.);
#4720=VECTOR('',#16557,10.);
#4721=VECTOR('',#16558,10.);
#4722=VECTOR('',#16559,10.);
#4723=VECTOR('',#16560,10.);
#4724=VECTOR('',#16561,10.);
#4725=VECTOR('',#16564,10.);
#4726=VECTOR('',#16565,10.);
#4727=VECTOR('',#16568,10.);
#4728=VECTOR('',#16575,10.);
#4729=VECTOR('',#16576,10.);
#4730=VECTOR('',#16577,10.);
#4731=VECTOR('',#16580,10.);
#4732=VECTOR('',#16587,10.);
#4733=VECTOR('',#16590,10.);
#4734=VECTOR('',#16595,10.);
#4735=VECTOR('',#16596,10.);
#4736=VECTOR('',#16603,10.);
#4737=VECTOR('',#16604,10.);
#4738=VECTOR('',#16609,10.);
#4739=VECTOR('',#16612,10.);
#4740=VECTOR('',#16615,10.);
#4741=VECTOR('',#16618,10.);
#4742=VECTOR('',#16621,10.);
#4743=VECTOR('',#16624,10.);
#4744=VECTOR('',#16629,10.);
#4745=VECTOR('',#16632,10.);
#4746=VECTOR('',#16637,10.);
#4747=VECTOR('',#16638,10.);
#4748=VECTOR('',#16639,10.);
#4749=VECTOR('',#16642,10.);
#4750=VECTOR('',#16643,10.);
#4751=VECTOR('',#16644,10.);
#4752=VECTOR('',#16647,10.);
#4753=VECTOR('',#16648,10.);
#4754=VECTOR('',#16651,10.);
#4755=VECTOR('',#16654,10.);
#4756=VECTOR('',#16657,10.);
#4757=VECTOR('',#16658,10.);
#4758=VECTOR('',#16661,10.);
#4759=VECTOR('',#16666,10.);
#4760=VECTOR('',#16667,10.);
#4761=VECTOR('',#16668,10.);
#4762=VECTOR('',#16671,10.);
#4763=VECTOR('',#16676,10.);
#4764=VECTOR('',#16677,10.);
#4765=VECTOR('',#16680,10.);
#4766=VECTOR('',#16685,10.);
#4767=VECTOR('',#16686,10.);
#4768=VECTOR('',#16689,10.);
#4769=VECTOR('',#16692,10.);
#4770=VECTOR('',#16693,10.);
#4771=VECTOR('',#16694,10.);
#4772=VECTOR('',#16695,10.);
#4773=VECTOR('',#16696,10.);
#4774=VECTOR('',#16697,10.);
#4775=VECTOR('',#16698,10.);
#4776=VECTOR('',#16699,10.);
#4777=VECTOR('',#16700,10.);
#4778=VECTOR('',#16701,10.);
#4779=VECTOR('',#16702,10.);
#4780=VECTOR('',#16703,10.);
#4781=VECTOR('',#16704,10.);
#4782=VECTOR('',#16705,10.);
#4783=VECTOR('',#16706,10.);
#4784=VECTOR('',#16707,10.);
#4785=VECTOR('',#16710,10.);
#4786=VECTOR('',#16711,10.);
#4787=VECTOR('',#16714,10.);
#4788=VECTOR('',#16721,10.);
#4789=VECTOR('',#16722,10.);
#4790=VECTOR('',#16723,10.);
#4791=VECTOR('',#16726,10.);
#4792=VECTOR('',#16731,10.);
#4793=VECTOR('',#16736,10.);
#4794=VECTOR('',#16737,10.);
#4795=VECTOR('',#16740,10.);
#4796=VECTOR('',#16745,10.);
#4797=VECTOR('',#16746,10.);
#4798=VECTOR('',#16749,10.);
#4799=VECTOR('',#16754,10.);
#4800=VECTOR('',#16759,10.);
#4801=VECTOR('',#16760,10.);
#4802=VECTOR('',#16761,10.);
#4803=VECTOR('',#16764,10.);
#4804=VECTOR('',#16765,10.);
#4805=VECTOR('',#16766,10.);
#4806=VECTOR('',#16769,10.);
#4807=VECTOR('',#16772,10.);
#4808=VECTOR('',#16775,10.);
#4809=VECTOR('',#16776,10.);
#4810=VECTOR('',#16777,10.);
#4811=VECTOR('',#16780,10.);
#4812=VECTOR('',#16781,10.);
#4813=VECTOR('',#16786,10.);
#4814=VECTOR('',#16787,10.);
#4815=VECTOR('',#16788,10.);
#4816=VECTOR('',#16791,10.);
#4817=VECTOR('',#16792,10.);
#4818=VECTOR('',#16793,10.);
#4819=VECTOR('',#16796,10.);
#4820=VECTOR('',#16799,10.);
#4821=VECTOR('',#16802,10.);
#4822=VECTOR('',#16803,10.);
#4823=VECTOR('',#16804,10.);
#4824=VECTOR('',#16807,10.);
#4825=VECTOR('',#16808,10.);
#4826=VECTOR('',#16813,10.);
#4827=VECTOR('',#16814,10.);
#4828=VECTOR('',#16815,10.);
#4829=VECTOR('',#16818,10.);
#4830=VECTOR('',#16819,10.);
#4831=VECTOR('',#16820,10.);
#4832=VECTOR('',#16823,10.);
#4833=VECTOR('',#16826,10.);
#4834=VECTOR('',#16829,10.);
#4835=VECTOR('',#16830,10.);
#4836=VECTOR('',#16831,10.);
#4837=VECTOR('',#16834,10.);
#4838=VECTOR('',#16835,10.);
#4839=VECTOR('',#16840,10.);
#4840=VECTOR('',#16841,10.);
#4841=VECTOR('',#16842,10.);
#4842=VECTOR('',#16845,10.);
#4843=VECTOR('',#16846,10.);
#4844=VECTOR('',#16847,10.);
#4845=VECTOR('',#16850,10.);
#4846=VECTOR('',#16853,10.);
#4847=VECTOR('',#16856,10.);
#4848=VECTOR('',#16857,10.);
#4849=VECTOR('',#16858,10.);
#4850=VECTOR('',#16861,10.);
#4851=VECTOR('',#16862,10.);
#4852=VECTOR('',#16867,1.525);
#4853=VECTOR('',#16872,1.525);
#4854=VECTOR('',#16877,1.525);
#4855=VECTOR('',#16882,1.525);
#4856=VECTOR('',#16887,1.525);
#4857=VECTOR('',#16890,10.);
#4858=VECTOR('',#16891,10.);
#4859=VECTOR('',#16894,10.);
#4860=VECTOR('',#16899,10.);
#4861=VECTOR('',#16900,10.);
#4862=VECTOR('',#16903,10.);
#4863=VECTOR('',#16908,10.);
#4864=VECTOR('',#16909,10.);
#4865=VECTOR('',#16912,10.);
#4866=VECTOR('',#16917,10.);
#4867=VECTOR('',#16918,10.);
#4868=VECTOR('',#16921,10.);
#4869=VECTOR('',#16926,10.);
#4870=VECTOR('',#16937,10.);
#6024=VERTEX_POINT('',#25939);
#6025=VERTEX_POINT('',#25940);
#6026=VERTEX_POINT('',#25944);
#6027=VERTEX_POINT('',#25946);
#6028=VERTEX_POINT('',#25950);
#6029=VERTEX_POINT('',#25952);
#6030=VERTEX_POINT('',#25956);
#6031=VERTEX_POINT('',#25957);
#6032=VERTEX_POINT('',#25964);
#6033=VERTEX_POINT('',#25966);
#6034=VERTEX_POINT('',#25968);
#6035=VERTEX_POINT('',#25970);
#6036=VERTEX_POINT('',#25972);
#6037=VERTEX_POINT('',#25976);
#6038=VERTEX_POINT('',#25979);
#6039=VERTEX_POINT('',#25982);
#6040=VERTEX_POINT('',#25984);
#6041=VERTEX_POINT('',#25986);
#6042=VERTEX_POINT('',#25988);
#6043=VERTEX_POINT('',#25992);
#6044=VERTEX_POINT('',#25994);
#6045=VERTEX_POINT('',#25998);
#6046=VERTEX_POINT('',#25999);
#6047=VERTEX_POINT('',#26001);
#6048=VERTEX_POINT('',#26003);
#6049=VERTEX_POINT('',#26005);
#6050=VERTEX_POINT('',#26007);
#6051=VERTEX_POINT('',#26009);
#6052=VERTEX_POINT('',#26011);
#6053=VERTEX_POINT('',#26015);
#6054=VERTEX_POINT('',#26019);
#6055=VERTEX_POINT('',#26020);
#6056=VERTEX_POINT('',#26024);
#6057=VERTEX_POINT('',#26026);
#6058=VERTEX_POINT('',#26030);
#6059=VERTEX_POINT('',#26032);
#6060=VERTEX_POINT('',#26036);
#6061=VERTEX_POINT('',#26037);
#6062=VERTEX_POINT('',#26044);
#6063=VERTEX_POINT('',#26046);
#6064=VERTEX_POINT('',#26048);
#6065=VERTEX_POINT('',#26050);
#6066=VERTEX_POINT('',#26052);
#6067=VERTEX_POINT('',#26056);
#6068=VERTEX_POINT('',#26059);
#6069=VERTEX_POINT('',#26062);
#6070=VERTEX_POINT('',#26064);
#6071=VERTEX_POINT('',#26066);
#6072=VERTEX_POINT('',#26068);
#6073=VERTEX_POINT('',#26072);
#6074=VERTEX_POINT('',#26074);
#6075=VERTEX_POINT('',#26078);
#6076=VERTEX_POINT('',#26079);
#6077=VERTEX_POINT('',#26084);
#6078=VERTEX_POINT('',#26085);
#6079=VERTEX_POINT('',#26090);
#6080=VERTEX_POINT('',#26091);
#6081=VERTEX_POINT('',#26099);
#6082=VERTEX_POINT('',#26101);
#6083=VERTEX_POINT('',#26103);
#6084=VERTEX_POINT('',#26105);
#6085=VERTEX_POINT('',#26107);
#6086=VERTEX_POINT('',#26109);
#6087=VERTEX_POINT('',#26111);
#6088=VERTEX_POINT('',#26116);
#6089=VERTEX_POINT('',#26120);
#6090=VERTEX_POINT('',#26124);
#6091=VERTEX_POINT('',#26129);
#6092=VERTEX_POINT('',#26131);
#6093=VERTEX_POINT('',#26133);
#6094=VERTEX_POINT('',#26135);
#6095=VERTEX_POINT('',#26137);
#6096=VERTEX_POINT('',#26139);
#6097=VERTEX_POINT('',#26143);
#6098=VERTEX_POINT('',#26147);
#6099=VERTEX_POINT('',#26148);
#6100=VERTEX_POINT('',#26153);
#6101=VERTEX_POINT('',#26154);
#6102=VERTEX_POINT('',#26159);
#6103=VERTEX_POINT('',#26166);
#6104=VERTEX_POINT('',#26170);
#6105=VERTEX_POINT('',#26177);
#6106=VERTEX_POINT('',#26191);
#6107=VERTEX_POINT('',#26197);
#6108=VERTEX_POINT('',#26201);
#6109=VERTEX_POINT('',#26203);
#6110=VERTEX_POINT('',#26207);
#6111=VERTEX_POINT('',#26209);
#6112=VERTEX_POINT('',#26216);
#6113=VERTEX_POINT('',#26218);
#6114=VERTEX_POINT('',#26222);
#6115=VERTEX_POINT('',#26226);
#6116=VERTEX_POINT('',#26230);
#6117=VERTEX_POINT('',#26235);
#6118=VERTEX_POINT('',#26239);
#6119=VERTEX_POINT('',#26243);
#6120=VERTEX_POINT('',#26252);
#6121=VERTEX_POINT('',#26253);
#6122=VERTEX_POINT('',#26255);
#6123=VERTEX_POINT('',#26257);
#6124=VERTEX_POINT('',#26260);
#6125=VERTEX_POINT('',#26261);
#6126=VERTEX_POINT('',#26263);
#6127=VERTEX_POINT('',#26265);
#6128=VERTEX_POINT('',#26268);
#6129=VERTEX_POINT('',#26269);
#6130=VERTEX_POINT('',#26271);
#6131=VERTEX_POINT('',#26273);
#6132=VERTEX_POINT('',#26276);
#6133=VERTEX_POINT('',#26277);
#6134=VERTEX_POINT('',#26279);
#6135=VERTEX_POINT('',#26281);
#6136=VERTEX_POINT('',#26285);
#6137=VERTEX_POINT('',#26289);
#6138=VERTEX_POINT('',#26290);
#6139=VERTEX_POINT('',#26295);
#6140=VERTEX_POINT('',#26300);
#6141=VERTEX_POINT('',#26307);
#6142=VERTEX_POINT('',#26311);
#6143=VERTEX_POINT('',#26315);
#6144=VERTEX_POINT('',#26319);
#6145=VERTEX_POINT('',#26326);
#6146=VERTEX_POINT('',#26328);
#6147=VERTEX_POINT('',#26332);
#6148=VERTEX_POINT('',#26334);
#6149=VERTEX_POINT('',#26342);
#6150=VERTEX_POINT('',#26344);
#6151=VERTEX_POINT('',#26348);
#6152=VERTEX_POINT('',#26351);
#6153=VERTEX_POINT('',#26354);
#6154=VERTEX_POINT('',#26356);
#6155=VERTEX_POINT('',#26360);
#6156=VERTEX_POINT('',#26362);
#6157=VERTEX_POINT('',#26370);
#6158=VERTEX_POINT('',#26372);
#6159=VERTEX_POINT('',#26376);
#6160=VERTEX_POINT('',#26379);
#6161=VERTEX_POINT('',#26382);
#6162=VERTEX_POINT('',#26384);
#6163=VERTEX_POINT('',#26388);
#6164=VERTEX_POINT('',#26390);
#6165=VERTEX_POINT('',#26398);
#6166=VERTEX_POINT('',#26400);
#6167=VERTEX_POINT('',#26404);
#6168=VERTEX_POINT('',#26407);
#6169=VERTEX_POINT('',#26410);
#6170=VERTEX_POINT('',#26412);
#6171=VERTEX_POINT('',#26416);
#6172=VERTEX_POINT('',#26418);
#6173=VERTEX_POINT('',#26426);
#6174=VERTEX_POINT('',#26428);
#6175=VERTEX_POINT('',#26432);
#6176=VERTEX_POINT('',#26435);
#6177=VERTEX_POINT('',#26438);
#6178=VERTEX_POINT('',#26442);
#6179=VERTEX_POINT('',#26446);
#6180=VERTEX_POINT('',#26450);
#6181=VERTEX_POINT('',#26456);
#6182=VERTEX_POINT('',#26463);
#6183=VERTEX_POINT('',#26470);
#6184=VERTEX_POINT('',#26477);
#7561=EDGE_CURVE('',#6024,#6025,#83,.F.);
#7562=EDGE_CURVE('',#6025,#6026,#951,.T.);
#7563=EDGE_CURVE('',#6026,#6027,#3355,.T.);
#7564=EDGE_CURVE('',#6027,#6024,#952,.T.);
#7565=EDGE_CURVE('',#6026,#6028,#3356,.T.);
#7566=EDGE_CURVE('',#6028,#6029,#3357,.T.);
#7567=EDGE_CURVE('',#6029,#6027,#3358,.T.);
#7568=EDGE_CURVE('',#6030,#6031,#84,.F.);
#7569=EDGE_CURVE('',#6031,#6029,#953,.T.);
#7570=EDGE_CURVE('',#6028,#6030,#954,.T.);
#7571=EDGE_CURVE('',#6032,#6030,#3359,.T.);
#7572=EDGE_CURVE('',#6028,#6033,#3360,.T.);
#7573=EDGE_CURVE('',#6034,#6033,#955,.T.);
#7574=EDGE_CURVE('',#6035,#6034,#3361,.T.);
#7575=EDGE_CURVE('',#6036,#6035,#956,.T.);
#7576=EDGE_CURVE('',#6032,#6036,#79,.F.);
#7577=EDGE_CURVE('',#6026,#6037,#3362,.T.);
#7578=EDGE_CURVE('',#6033,#6037,#3363,.T.);
#7579=EDGE_CURVE('',#6038,#6038,#957,.T.);
#7580=EDGE_CURVE('',#6025,#6039,#3364,.T.);
#7581=EDGE_CURVE('',#6039,#6040,#80,.T.);
#7582=EDGE_CURVE('',#6041,#6040,#958,.T.);
#7583=EDGE_CURVE('',#6041,#6042,#3365,.T.);
#7584=EDGE_CURVE('',#6037,#6042,#959,.T.);
#7585=EDGE_CURVE('',#6043,#6043,#960,.T.);
#7586=EDGE_CURVE('',#6043,#6044,#3366,.T.);
#7587=EDGE_CURVE('',#6044,#6044,#961,.T.);
#7588=EDGE_CURVE('',#6045,#6046,#962,.T.);
#7589=EDGE_CURVE('',#6047,#6045,#3367,.T.);
#7590=EDGE_CURVE('',#6048,#6047,#963,.T.);
#7591=EDGE_CURVE('',#6049,#6048,#3368,.T.);
#7592=EDGE_CURVE('',#6050,#6049,#964,.T.);
#7593=EDGE_CURVE('',#6051,#6050,#3369,.T.);
#7594=EDGE_CURVE('',#6052,#6051,#965,.T.);
#7595=EDGE_CURVE('',#6046,#6052,#3370,.T.);
#7596=EDGE_CURVE('',#6044,#6053,#3371,.T.);
#7597=EDGE_CURVE('',#6053,#6053,#966,.T.);
#7598=EDGE_CURVE('',#6054,#6055,#85,.F.);
#7599=EDGE_CURVE('',#6055,#6056,#967,.T.);
#7600=EDGE_CURVE('',#6056,#6057,#3372,.T.);
#7601=EDGE_CURVE('',#6057,#6054,#968,.T.);
#7602=EDGE_CURVE('',#6056,#6058,#3373,.T.);
#7603=EDGE_CURVE('',#6058,#6059,#3374,.T.);
#7604=EDGE_CURVE('',#6059,#6057,#3375,.T.);
#7605=EDGE_CURVE('',#6060,#6061,#86,.F.);
#7606=EDGE_CURVE('',#6061,#6059,#969,.T.);
#7607=EDGE_CURVE('',#6058,#6060,#970,.T.);
#7608=EDGE_CURVE('',#6062,#6060,#3376,.T.);
#7609=EDGE_CURVE('',#6058,#6063,#3377,.T.);
#7610=EDGE_CURVE('',#6064,#6063,#971,.T.);
#7611=EDGE_CURVE('',#6065,#6064,#3378,.T.);
#7612=EDGE_CURVE('',#6066,#6065,#972,.T.);
#7613=EDGE_CURVE('',#6062,#6066,#81,.F.);
#7614=EDGE_CURVE('',#6056,#6067,#3379,.T.);
#7615=EDGE_CURVE('',#6063,#6067,#3380,.T.);
#7616=EDGE_CURVE('',#6068,#6068,#973,.T.);
#7617=EDGE_CURVE('',#6055,#6069,#3381,.T.);
#7618=EDGE_CURVE('',#6069,#6070,#82,.T.);
#7619=EDGE_CURVE('',#6071,#6070,#974,.T.);
#7620=EDGE_CURVE('',#6071,#6072,#3382,.T.);
#7621=EDGE_CURVE('',#6067,#6072,#975,.T.);
#7622=EDGE_CURVE('',#6069,#6073,#3383,.T.);
#7623=EDGE_CURVE('',#6073,#6074,#3384,.T.);
#7624=EDGE_CURVE('',#6074,#6070,#3385,.T.);
#7625=EDGE_CURVE('',#6075,#6076,#3386,.T.);
#7626=EDGE_CURVE('',#6076,#6074,#976,.T.);
#7627=EDGE_CURVE('',#6073,#6075,#977,.T.);
#7628=EDGE_CURVE('',#6077,#6078,#3387,.T.);
#7629=EDGE_CURVE('',#6078,#6076,#3388,.T.);
#7630=EDGE_CURVE('',#6075,#6077,#3389,.T.);
#7631=EDGE_CURVE('',#6079,#6080,#3390,.T.);
#7632=EDGE_CURVE('',#6080,#6078,#978,.T.);
#7633=EDGE_CURVE('',#6077,#6079,#979,.T.);
#7634=EDGE_CURVE('',#6036,#6080,#3391,.T.);
#7635=EDGE_CURVE('',#6079,#6032,#3392,.T.);
#7636=EDGE_CURVE('',#6081,#6079,#3393,.T.);
#7637=EDGE_CURVE('',#6082,#6081,#3394,.T.);
#7638=EDGE_CURVE('',#6082,#6083,#3395,.T.);
#7639=EDGE_CURVE('',#6084,#6083,#3396,.T.);
#7640=EDGE_CURVE('',#6085,#6084,#3397,.T.);
#7641=EDGE_CURVE('',#6086,#6085,#3398,.T.);
#7642=EDGE_CURVE('',#6086,#6087,#3399,.T.);
#7643=EDGE_CURVE('',#6039,#6087,#3400,.T.);
#7644=EDGE_CURVE('',#6031,#6024,#3401,.T.);
#7645=EDGE_CURVE('',#6088,#6077,#3402,.T.);
#7646=EDGE_CURVE('',#6081,#6088,#980,.T.);
#7647=EDGE_CURVE('',#6089,#6075,#3403,.T.);
#7648=EDGE_CURVE('',#6088,#6089,#3404,.T.);
#7649=EDGE_CURVE('',#6090,#6073,#3405,.T.);
#7650=EDGE_CURVE('',#6089,#6090,#981,.T.);
#7651=EDGE_CURVE('',#6061,#6054,#3406,.T.);
#7652=EDGE_CURVE('',#6091,#6062,#3407,.T.);
#7653=EDGE_CURVE('',#6092,#6091,#3408,.T.);
#7654=EDGE_CURVE('',#6093,#6092,#3409,.T.);
#7655=EDGE_CURVE('',#6094,#6093,#3410,.T.);
#7656=EDGE_CURVE('',#6095,#6094,#3411,.T.);
#7657=EDGE_CURVE('',#6096,#6095,#3412,.T.);
#7658=EDGE_CURVE('',#6090,#6096,#3413,.T.);
#7659=EDGE_CURVE('',#6087,#6097,#3414,.T.);
#7660=EDGE_CURVE('',#6097,#6040,#3415,.T.);
#7661=EDGE_CURVE('',#6098,#6099,#3416,.T.);
#7662=EDGE_CURVE('',#6099,#6097,#982,.T.);
#7663=EDGE_CURVE('',#6087,#6098,#983,.T.);
#7664=EDGE_CURVE('',#6100,#6101,#3417,.T.);
#7665=EDGE_CURVE('',#6101,#6099,#3418,.T.);
#7666=EDGE_CURVE('',#6098,#6100,#3419,.T.);
#7667=EDGE_CURVE('',#6091,#6102,#3420,.T.);
#7668=EDGE_CURVE('',#6102,#6101,#984,.T.);
#7669=EDGE_CURVE('',#6100,#6091,#985,.T.);
#7670=EDGE_CURVE('',#6066,#6102,#3421,.T.);
#7671=EDGE_CURVE('',#6103,#6100,#3422,.T.);
#7672=EDGE_CURVE('',#6092,#6103,#986,.T.);
#7673=EDGE_CURVE('',#6104,#6098,#3423,.T.);
#7674=EDGE_CURVE('',#6103,#6104,#3424,.T.);
#7675=EDGE_CURVE('',#6104,#6086,#987,.T.);
#7676=EDGE_CURVE('',#6082,#6045,#3425,.T.);
#7677=EDGE_CURVE('',#6046,#6105,#3426,.T.);
#7678=EDGE_CURVE('',#6105,#6082,#988,.T.);
#7679=EDGE_CURVE('',#6081,#6047,#3427,.T.);
#7680=EDGE_CURVE('',#6088,#6048,#3428,.T.);
#7681=EDGE_CURVE('',#6089,#6049,#3429,.T.);
#7682=EDGE_CURVE('',#6090,#6050,#3430,.T.);
#7683=EDGE_CURVE('',#6096,#6051,#3431,.T.);
#7684=EDGE_CURVE('',#6106,#6052,#3432,.T.);
#7685=EDGE_CURVE('',#6096,#6106,#989,.T.);
#7686=EDGE_CURVE('',#6106,#6105,#3433,.T.);
#7687=EDGE_CURVE('',#6105,#6107,#3434,.T.);
#7688=EDGE_CURVE('',#6083,#6107,#990,.T.);
#7689=EDGE_CURVE('',#6093,#6108,#3435,.F.);
#7690=EDGE_CURVE('',#6108,#6109,#3436,.T.);
#7691=EDGE_CURVE('',#6109,#6094,#3437,.F.);
#7692=EDGE_CURVE('',#6110,#6108,#3438,.T.);
#7693=EDGE_CURVE('',#6111,#6110,#3439,.T.);
#7694=EDGE_CURVE('',#6109,#6111,#3440,.T.);
#7695=EDGE_CURVE('',#6084,#6111,#3441,.F.);
#7696=EDGE_CURVE('',#6110,#6085,#3442,.F.);
#7697=EDGE_CURVE('',#6033,#6112,#3443,.T.);
#7698=EDGE_CURVE('',#6112,#6113,#991,.T.);
#7699=EDGE_CURVE('',#6113,#6034,#3444,.T.);
#7700=EDGE_CURVE('',#6037,#6114,#3445,.T.);
#7701=EDGE_CURVE('',#6114,#6112,#3446,.T.);
#7702=EDGE_CURVE('',#6042,#6115,#3447,.T.);
#7703=EDGE_CURVE('',#6115,#6114,#992,.T.);
#7704=EDGE_CURVE('',#6064,#6116,#3448,.T.);
#7705=EDGE_CURVE('',#6116,#6115,#3449,.T.);
#7706=EDGE_CURVE('',#6042,#6064,#3450,.T.);
#7707=EDGE_CURVE('',#6063,#6117,#3451,.T.);
#7708=EDGE_CURVE('',#6117,#6116,#993,.T.);
#7709=EDGE_CURVE('',#6067,#6118,#3452,.T.);
#7710=EDGE_CURVE('',#6118,#6117,#3453,.T.);
#7711=EDGE_CURVE('',#6072,#6119,#3454,.T.);
#7712=EDGE_CURVE('',#6119,#6118,#994,.T.);
#7713=EDGE_CURVE('',#6113,#6119,#3455,.T.);
#7714=EDGE_CURVE('',#6072,#6034,#3456,.T.);
#7715=EDGE_CURVE('',#6065,#6041,#3457,.T.);
#7716=EDGE_CURVE('',#6120,#6121,#3458,.T.);
#7717=EDGE_CURVE('',#6122,#6120,#3459,.T.);
#7718=EDGE_CURVE('',#6123,#6122,#3460,.T.);
#7719=EDGE_CURVE('',#6121,#6123,#3461,.T.);
#7720=EDGE_CURVE('',#6124,#6125,#3462,.T.);
#7721=EDGE_CURVE('',#6126,#6124,#3463,.T.);
#7722=EDGE_CURVE('',#6127,#6126,#3464,.T.);
#7723=EDGE_CURVE('',#6125,#6127,#3465,.T.);
#7724=EDGE_CURVE('',#6128,#6129,#3466,.T.);
#7725=EDGE_CURVE('',#6130,#6128,#3467,.T.);
#7726=EDGE_CURVE('',#6131,#6130,#3468,.T.);
#7727=EDGE_CURVE('',#6129,#6131,#3469,.T.);
#7728=EDGE_CURVE('',#6132,#6133,#3470,.T.);
#7729=EDGE_CURVE('',#6134,#6132,#3471,.T.);
#7730=EDGE_CURVE('',#6135,#6134,#3472,.T.);
#7731=EDGE_CURVE('',#6133,#6135,#3473,.T.);
#7732=EDGE_CURVE('',#6109,#6136,#3474,.T.);
#7733=EDGE_CURVE('',#6136,#6095,#3475,.T.);
#7734=EDGE_CURVE('',#6137,#6138,#3476,.T.);
#7735=EDGE_CURVE('',#6138,#6095,#995,.T.);
#7736=EDGE_CURVE('',#6136,#6137,#996,.T.);
#7737=EDGE_CURVE('',#6139,#6107,#3477,.T.);
#7738=EDGE_CURVE('',#6107,#6138,#3478,.T.);
#7739=EDGE_CURVE('',#6137,#6139,#3479,.T.);
#7740=EDGE_CURVE('',#6140,#6083,#3480,.T.);
#7741=EDGE_CURVE('',#6139,#6140,#997,.T.);
#7742=EDGE_CURVE('',#6140,#6111,#3481,.T.);
#7743=EDGE_CURVE('',#6110,#6141,#3482,.T.);
#7744=EDGE_CURVE('',#6141,#6086,#3483,.T.);
#7745=EDGE_CURVE('',#6142,#6104,#3484,.T.);
#7746=EDGE_CURVE('',#6141,#6142,#998,.T.);
#7747=EDGE_CURVE('',#6143,#6103,#3485,.T.);
#7748=EDGE_CURVE('',#6142,#6143,#3486,.T.);
#7749=EDGE_CURVE('',#6144,#6092,#3487,.T.);
#7750=EDGE_CURVE('',#6143,#6144,#999,.T.);
#7751=EDGE_CURVE('',#6144,#6108,#3488,.T.);
#7752=EDGE_CURVE('',#6122,#6145,#3489,.T.);
#7753=EDGE_CURVE('',#6145,#6146,#3490,.T.);
#7754=EDGE_CURVE('',#6123,#6146,#3491,.T.);
#7755=EDGE_CURVE('',#6121,#6147,#3492,.T.);
#7756=EDGE_CURVE('',#6147,#6148,#3493,.T.);
#7757=EDGE_CURVE('',#6148,#6120,#3494,.T.);
#7758=EDGE_CURVE('',#6146,#6147,#3495,.T.);
#7759=EDGE_CURVE('',#6148,#6145,#3496,.T.);
#7760=EDGE_CURVE('',#6148,#6149,#3497,.T.);
#7761=EDGE_CURVE('',#6149,#6150,#3498,.T.);
#7762=EDGE_CURVE('',#6145,#6150,#3499,.T.);
#7763=EDGE_CURVE('',#6147,#6151,#3500,.T.);
#7764=EDGE_CURVE('',#6151,#6149,#3501,.T.);
#7765=EDGE_CURVE('',#6152,#6152,#1000,.T.);
#7766=EDGE_CURVE('',#6134,#6153,#3502,.T.);
#7767=EDGE_CURVE('',#6153,#6154,#3503,.T.);
#7768=EDGE_CURVE('',#6135,#6154,#3504,.T.);
#7769=EDGE_CURVE('',#6133,#6155,#3505,.T.);
#7770=EDGE_CURVE('',#6155,#6156,#3506,.T.);
#7771=EDGE_CURVE('',#6156,#6132,#3507,.T.);
#7772=EDGE_CURVE('',#6154,#6155,#3508,.T.);
#7773=EDGE_CURVE('',#6156,#6153,#3509,.T.);
#7774=EDGE_CURVE('',#6156,#6157,#3510,.T.);
#7775=EDGE_CURVE('',#6157,#6158,#3511,.T.);
#7776=EDGE_CURVE('',#6153,#6158,#3512,.T.);
#7777=EDGE_CURVE('',#6155,#6159,#3513,.T.);
#7778=EDGE_CURVE('',#6159,#6157,#3514,.T.);
#7779=EDGE_CURVE('',#6160,#6160,#1001,.T.);
#7780=EDGE_CURVE('',#6126,#6161,#3515,.T.);
#7781=EDGE_CURVE('',#6161,#6162,#3516,.T.);
#7782=EDGE_CURVE('',#6127,#6162,#3517,.T.);
#7783=EDGE_CURVE('',#6125,#6163,#3518,.T.);
#7784=EDGE_CURVE('',#6163,#6164,#3519,.T.);
#7785=EDGE_CURVE('',#6164,#6124,#3520,.T.);
#7786=EDGE_CURVE('',#6162,#6163,#3521,.T.);
#7787=EDGE_CURVE('',#6164,#6161,#3522,.T.);
#7788=EDGE_CURVE('',#6164,#6165,#3523,.T.);
#7789=EDGE_CURVE('',#6165,#6166,#3524,.T.);
#7790=EDGE_CURVE('',#6161,#6166,#3525,.T.);
#7791=EDGE_CURVE('',#6163,#6167,#3526,.T.);
#7792=EDGE_CURVE('',#6167,#6165,#3527,.T.);
#7793=EDGE_CURVE('',#6168,#6168,#1002,.T.);
#7794=EDGE_CURVE('',#6130,#6169,#3528,.T.);
#7795=EDGE_CURVE('',#6169,#6170,#3529,.T.);
#7796=EDGE_CURVE('',#6131,#6170,#3530,.T.);
#7797=EDGE_CURVE('',#6129,#6171,#3531,.T.);
#7798=EDGE_CURVE('',#6171,#6172,#3532,.T.);
#7799=EDGE_CURVE('',#6172,#6128,#3533,.T.);
#7800=EDGE_CURVE('',#6170,#6171,#3534,.T.);
#7801=EDGE_CURVE('',#6172,#6169,#3535,.T.);
#7802=EDGE_CURVE('',#6172,#6173,#3536,.T.);
#7803=EDGE_CURVE('',#6173,#6174,#3537,.T.);
#7804=EDGE_CURVE('',#6169,#6174,#3538,.T.);
#7805=EDGE_CURVE('',#6171,#6175,#3539,.T.);
#7806=EDGE_CURVE('',#6175,#6173,#3540,.T.);
#7807=EDGE_CURVE('',#6176,#6176,#1003,.T.);
#7808=EDGE_CURVE('',#6038,#6177,#3541,.T.);
#7809=EDGE_CURVE('',#6177,#6177,#1004,.T.);
#7810=EDGE_CURVE('',#6168,#6178,#3542,.T.);
#7811=EDGE_CURVE('',#6178,#6178,#1005,.T.);
#7812=EDGE_CURVE('',#6176,#6179,#3543,.T.);
#7813=EDGE_CURVE('',#6179,#6179,#1006,.T.);
#7814=EDGE_CURVE('',#6152,#6180,#3544,.T.);
#7815=EDGE_CURVE('',#6180,#6180,#1007,.T.);
#7816=EDGE_CURVE('',#6160,#6068,#3545,.T.);
#7817=EDGE_CURVE('',#6170,#6181,#3546,.T.);
#7818=EDGE_CURVE('',#6181,#6175,#3547,.T.);
#7819=EDGE_CURVE('',#6174,#6181,#3548,.T.);
#7820=EDGE_CURVE('',#6162,#6182,#3549,.T.);
#7821=EDGE_CURVE('',#6182,#6167,#3550,.T.);
#7822=EDGE_CURVE('',#6166,#6182,#3551,.T.);
#7823=EDGE_CURVE('',#6154,#6183,#3552,.T.);
#7824=EDGE_CURVE('',#6183,#6159,#3553,.T.);
#7825=EDGE_CURVE('',#6158,#6183,#3554,.T.);
#7826=EDGE_CURVE('',#6146,#6184,#3555,.T.);
#7827=EDGE_CURVE('',#6184,#6151,#3556,.T.);
#7828=EDGE_CURVE('',#6150,#6184,#3557,.T.);
#7829=EDGE_CURVE('',#6106,#6138,#3558,.T.);
#7830=EDGE_CURVE('',#6035,#6071,#3559,.T.);
#10369=ORIENTED_EDGE('',*,*,#7561,.T.);
#10370=ORIENTED_EDGE('',*,*,#7562,.T.);
#10371=ORIENTED_EDGE('',*,*,#7563,.T.);
#10372=ORIENTED_EDGE('',*,*,#7564,.T.);
#10373=ORIENTED_EDGE('',*,*,#7563,.F.);
#10374=ORIENTED_EDGE('',*,*,#7565,.T.);
#10375=ORIENTED_EDGE('',*,*,#7566,.T.);
#10376=ORIENTED_EDGE('',*,*,#7567,.T.);
#10377=ORIENTED_EDGE('',*,*,#7568,.T.);
#10378=ORIENTED_EDGE('',*,*,#7569,.T.);
#10379=ORIENTED_EDGE('',*,*,#7566,.F.);
#10380=ORIENTED_EDGE('',*,*,#7570,.T.);
#10381=ORIENTED_EDGE('',*,*,#7571,.T.);
#10382=ORIENTED_EDGE('',*,*,#7570,.F.);
#10383=ORIENTED_EDGE('',*,*,#7572,.T.);
#10384=ORIENTED_EDGE('',*,*,#7573,.F.);
#10385=ORIENTED_EDGE('',*,*,#7574,.F.);
#10386=ORIENTED_EDGE('',*,*,#7575,.F.);
#10387=ORIENTED_EDGE('',*,*,#7576,.F.);
#10388=ORIENTED_EDGE('',*,*,#7565,.F.);
#10389=ORIENTED_EDGE('',*,*,#7577,.T.);
#10390=ORIENTED_EDGE('',*,*,#7578,.F.);
#10391=ORIENTED_EDGE('',*,*,#7572,.F.);
#10392=ORIENTED_EDGE('',*,*,#7579,.T.);
#10393=ORIENTED_EDGE('',*,*,#7562,.F.);
#10394=ORIENTED_EDGE('',*,*,#7580,.T.);
#10395=ORIENTED_EDGE('',*,*,#7581,.T.);
#10396=ORIENTED_EDGE('',*,*,#7582,.F.);
#10397=ORIENTED_EDGE('',*,*,#7583,.T.);
#10398=ORIENTED_EDGE('',*,*,#7584,.F.);
#10399=ORIENTED_EDGE('',*,*,#7577,.F.);
#10400=ORIENTED_EDGE('',*,*,#7585,.T.);
#10401=ORIENTED_EDGE('',*,*,#7586,.T.);
#10402=ORIENTED_EDGE('',*,*,#7587,.T.);
#10403=ORIENTED_EDGE('',*,*,#7586,.F.);
#10404=ORIENTED_EDGE('',*,*,#7588,.F.);
#10405=ORIENTED_EDGE('',*,*,#7589,.F.);
#10406=ORIENTED_EDGE('',*,*,#7590,.F.);
#10407=ORIENTED_EDGE('',*,*,#7591,.F.);
#10408=ORIENTED_EDGE('',*,*,#7592,.F.);
#10409=ORIENTED_EDGE('',*,*,#7593,.F.);
#10410=ORIENTED_EDGE('',*,*,#7594,.F.);
#10411=ORIENTED_EDGE('',*,*,#7595,.F.);
#10412=ORIENTED_EDGE('',*,*,#7585,.F.);
#10413=ORIENTED_EDGE('',*,*,#7587,.F.);
#10414=ORIENTED_EDGE('',*,*,#7596,.T.);
#10415=ORIENTED_EDGE('',*,*,#7597,.T.);
#10416=ORIENTED_EDGE('',*,*,#7596,.F.);
#10417=ORIENTED_EDGE('',*,*,#7598,.T.);
#10418=ORIENTED_EDGE('',*,*,#7599,.T.);
#10419=ORIENTED_EDGE('',*,*,#7600,.T.);
#10420=ORIENTED_EDGE('',*,*,#7601,.T.);
#10421=ORIENTED_EDGE('',*,*,#7600,.F.);
#10422=ORIENTED_EDGE('',*,*,#7602,.T.);
#10423=ORIENTED_EDGE('',*,*,#7603,.T.);
#10424=ORIENTED_EDGE('',*,*,#7604,.T.);
#10425=ORIENTED_EDGE('',*,*,#7605,.T.);
#10426=ORIENTED_EDGE('',*,*,#7606,.T.);
#10427=ORIENTED_EDGE('',*,*,#7603,.F.);
#10428=ORIENTED_EDGE('',*,*,#7607,.T.);
#10429=ORIENTED_EDGE('',*,*,#7608,.T.);
#10430=ORIENTED_EDGE('',*,*,#7607,.F.);
#10431=ORIENTED_EDGE('',*,*,#7609,.T.);
#10432=ORIENTED_EDGE('',*,*,#7610,.F.);
#10433=ORIENTED_EDGE('',*,*,#7611,.F.);
#10434=ORIENTED_EDGE('',*,*,#7612,.F.);
#10435=ORIENTED_EDGE('',*,*,#7613,.F.);
#10436=ORIENTED_EDGE('',*,*,#7602,.F.);
#10437=ORIENTED_EDGE('',*,*,#7614,.T.);
#10438=ORIENTED_EDGE('',*,*,#7615,.F.);
#10439=ORIENTED_EDGE('',*,*,#7609,.F.);
#10440=ORIENTED_EDGE('',*,*,#7616,.T.);
#10441=ORIENTED_EDGE('',*,*,#7599,.F.);
#10442=ORIENTED_EDGE('',*,*,#7617,.T.);
#10443=ORIENTED_EDGE('',*,*,#7618,.T.);
#10444=ORIENTED_EDGE('',*,*,#7619,.F.);
#10445=ORIENTED_EDGE('',*,*,#7620,.T.);
#10446=ORIENTED_EDGE('',*,*,#7621,.F.);
#10447=ORIENTED_EDGE('',*,*,#7614,.F.);
#10448=ORIENTED_EDGE('',*,*,#7618,.F.);
#10449=ORIENTED_EDGE('',*,*,#7622,.T.);
#10450=ORIENTED_EDGE('',*,*,#7623,.T.);
#10451=ORIENTED_EDGE('',*,*,#7624,.T.);
#10452=ORIENTED_EDGE('',*,*,#7625,.T.);
#10453=ORIENTED_EDGE('',*,*,#7626,.T.);
#10454=ORIENTED_EDGE('',*,*,#7623,.F.);
#10455=ORIENTED_EDGE('',*,*,#7627,.T.);
#10456=ORIENTED_EDGE('',*,*,#7628,.T.);
#10457=ORIENTED_EDGE('',*,*,#7629,.T.);
#10458=ORIENTED_EDGE('',*,*,#7625,.F.);
#10459=ORIENTED_EDGE('',*,*,#7630,.T.);
#10460=ORIENTED_EDGE('',*,*,#7631,.T.);
#10461=ORIENTED_EDGE('',*,*,#7632,.T.);
#10462=ORIENTED_EDGE('',*,*,#7628,.F.);
#10463=ORIENTED_EDGE('',*,*,#7633,.T.);
#10464=ORIENTED_EDGE('',*,*,#7576,.T.);
#10465=ORIENTED_EDGE('',*,*,#7634,.T.);
#10466=ORIENTED_EDGE('',*,*,#7631,.F.);
#10467=ORIENTED_EDGE('',*,*,#7635,.T.);
#10468=ORIENTED_EDGE('',*,*,#7571,.F.);
#10469=ORIENTED_EDGE('',*,*,#7635,.F.);
#10470=ORIENTED_EDGE('',*,*,#7636,.F.);
#10471=ORIENTED_EDGE('',*,*,#7637,.F.);
#10472=ORIENTED_EDGE('',*,*,#7638,.T.);
#10473=ORIENTED_EDGE('',*,*,#7639,.F.);
#10474=ORIENTED_EDGE('',*,*,#7640,.F.);
#10475=ORIENTED_EDGE('',*,*,#7641,.F.);
#10476=ORIENTED_EDGE('',*,*,#7642,.T.);
#10477=ORIENTED_EDGE('',*,*,#7643,.F.);
#10478=ORIENTED_EDGE('',*,*,#7580,.F.);
#10479=ORIENTED_EDGE('',*,*,#7561,.F.);
#10480=ORIENTED_EDGE('',*,*,#7644,.F.);
#10481=ORIENTED_EDGE('',*,*,#7568,.F.);
#10482=ORIENTED_EDGE('',*,*,#7633,.F.);
#10483=ORIENTED_EDGE('',*,*,#7645,.F.);
#10484=ORIENTED_EDGE('',*,*,#7646,.F.);
#10485=ORIENTED_EDGE('',*,*,#7636,.T.);
#10486=ORIENTED_EDGE('',*,*,#7630,.F.);
#10487=ORIENTED_EDGE('',*,*,#7647,.F.);
#10488=ORIENTED_EDGE('',*,*,#7648,.F.);
#10489=ORIENTED_EDGE('',*,*,#7645,.T.);
#10490=ORIENTED_EDGE('',*,*,#7627,.F.);
#10491=ORIENTED_EDGE('',*,*,#7649,.F.);
#10492=ORIENTED_EDGE('',*,*,#7650,.F.);
#10493=ORIENTED_EDGE('',*,*,#7647,.T.);
#10494=ORIENTED_EDGE('',*,*,#7622,.F.);
#10495=ORIENTED_EDGE('',*,*,#7617,.F.);
#10496=ORIENTED_EDGE('',*,*,#7598,.F.);
#10497=ORIENTED_EDGE('',*,*,#7651,.F.);
#10498=ORIENTED_EDGE('',*,*,#7605,.F.);
#10499=ORIENTED_EDGE('',*,*,#7608,.F.);
#10500=ORIENTED_EDGE('',*,*,#7652,.F.);
#10501=ORIENTED_EDGE('',*,*,#7653,.F.);
#10502=ORIENTED_EDGE('',*,*,#7654,.F.);
#10503=ORIENTED_EDGE('',*,*,#7655,.F.);
#10504=ORIENTED_EDGE('',*,*,#7656,.F.);
#10505=ORIENTED_EDGE('',*,*,#7657,.F.);
#10506=ORIENTED_EDGE('',*,*,#7658,.F.);
#10507=ORIENTED_EDGE('',*,*,#7649,.T.);
#10508=ORIENTED_EDGE('',*,*,#7581,.F.);
#10509=ORIENTED_EDGE('',*,*,#7643,.T.);
#10510=ORIENTED_EDGE('',*,*,#7659,.T.);
#10511=ORIENTED_EDGE('',*,*,#7660,.T.);
#10512=ORIENTED_EDGE('',*,*,#7661,.T.);
#10513=ORIENTED_EDGE('',*,*,#7662,.T.);
#10514=ORIENTED_EDGE('',*,*,#7659,.F.);
#10515=ORIENTED_EDGE('',*,*,#7663,.T.);
#10516=ORIENTED_EDGE('',*,*,#7664,.T.);
#10517=ORIENTED_EDGE('',*,*,#7665,.T.);
#10518=ORIENTED_EDGE('',*,*,#7661,.F.);
#10519=ORIENTED_EDGE('',*,*,#7666,.T.);
#10520=ORIENTED_EDGE('',*,*,#7667,.T.);
#10521=ORIENTED_EDGE('',*,*,#7668,.T.);
#10522=ORIENTED_EDGE('',*,*,#7664,.F.);
#10523=ORIENTED_EDGE('',*,*,#7669,.T.);
#10524=ORIENTED_EDGE('',*,*,#7613,.T.);
#10525=ORIENTED_EDGE('',*,*,#7670,.T.);
#10526=ORIENTED_EDGE('',*,*,#7667,.F.);
#10527=ORIENTED_EDGE('',*,*,#7652,.T.);
#10528=ORIENTED_EDGE('',*,*,#7669,.F.);
#10529=ORIENTED_EDGE('',*,*,#7671,.F.);
#10530=ORIENTED_EDGE('',*,*,#7672,.F.);
#10531=ORIENTED_EDGE('',*,*,#7653,.T.);
#10532=ORIENTED_EDGE('',*,*,#7666,.F.);
#10533=ORIENTED_EDGE('',*,*,#7673,.F.);
#10534=ORIENTED_EDGE('',*,*,#7674,.F.);
#10535=ORIENTED_EDGE('',*,*,#7671,.T.);
#10536=ORIENTED_EDGE('',*,*,#7663,.F.);
#10537=ORIENTED_EDGE('',*,*,#7642,.F.);
#10538=ORIENTED_EDGE('',*,*,#7675,.F.);
#10539=ORIENTED_EDGE('',*,*,#7673,.T.);
#10540=ORIENTED_EDGE('',*,*,#7676,.T.);
#10541=ORIENTED_EDGE('',*,*,#7588,.T.);
#10542=ORIENTED_EDGE('',*,*,#7677,.T.);
#10543=ORIENTED_EDGE('',*,*,#7678,.T.);
#10544=ORIENTED_EDGE('',*,*,#7676,.F.);
#10545=ORIENTED_EDGE('',*,*,#7637,.T.);
#10546=ORIENTED_EDGE('',*,*,#7679,.T.);
#10547=ORIENTED_EDGE('',*,*,#7589,.T.);
#10548=ORIENTED_EDGE('',*,*,#7680,.T.);
#10549=ORIENTED_EDGE('',*,*,#7590,.T.);
#10550=ORIENTED_EDGE('',*,*,#7679,.F.);
#10551=ORIENTED_EDGE('',*,*,#7646,.T.);
#10552=ORIENTED_EDGE('',*,*,#7680,.F.);
#10553=ORIENTED_EDGE('',*,*,#7648,.T.);
#10554=ORIENTED_EDGE('',*,*,#7681,.T.);
#10555=ORIENTED_EDGE('',*,*,#7591,.T.);
#10556=ORIENTED_EDGE('',*,*,#7682,.T.);
#10557=ORIENTED_EDGE('',*,*,#7592,.T.);
#10558=ORIENTED_EDGE('',*,*,#7681,.F.);
#10559=ORIENTED_EDGE('',*,*,#7650,.T.);
#10560=ORIENTED_EDGE('',*,*,#7682,.F.);
#10561=ORIENTED_EDGE('',*,*,#7658,.T.);
#10562=ORIENTED_EDGE('',*,*,#7683,.T.);
#10563=ORIENTED_EDGE('',*,*,#7593,.T.);
#10564=ORIENTED_EDGE('',*,*,#7684,.T.);
#10565=ORIENTED_EDGE('',*,*,#7594,.T.);
#10566=ORIENTED_EDGE('',*,*,#7683,.F.);
#10567=ORIENTED_EDGE('',*,*,#7685,.T.);
#10568=ORIENTED_EDGE('',*,*,#7684,.F.);
#10569=ORIENTED_EDGE('',*,*,#7686,.T.);
#10570=ORIENTED_EDGE('',*,*,#7677,.F.);
#10571=ORIENTED_EDGE('',*,*,#7595,.T.);
#10572=ORIENTED_EDGE('',*,*,#7678,.F.);
#10573=ORIENTED_EDGE('',*,*,#7687,.T.);
#10574=ORIENTED_EDGE('',*,*,#7688,.F.);
#10575=ORIENTED_EDGE('',*,*,#7638,.F.);
#10576=ORIENTED_EDGE('',*,*,#7689,.T.);
#10577=ORIENTED_EDGE('',*,*,#7690,.T.);
#10578=ORIENTED_EDGE('',*,*,#7691,.T.);
#10579=ORIENTED_EDGE('',*,*,#7655,.T.);
#10580=ORIENTED_EDGE('',*,*,#7690,.F.);
#10581=ORIENTED_EDGE('',*,*,#7692,.F.);
#10582=ORIENTED_EDGE('',*,*,#7693,.F.);
#10583=ORIENTED_EDGE('',*,*,#7694,.F.);
#10584=ORIENTED_EDGE('',*,*,#7695,.T.);
#10585=ORIENTED_EDGE('',*,*,#7693,.T.);
#10586=ORIENTED_EDGE('',*,*,#7696,.T.);
#10587=ORIENTED_EDGE('',*,*,#7640,.T.);
#10588=ORIENTED_EDGE('',*,*,#7697,.T.);
#10589=ORIENTED_EDGE('',*,*,#7698,.T.);
#10590=ORIENTED_EDGE('',*,*,#7699,.T.);
#10591=ORIENTED_EDGE('',*,*,#7573,.T.);
#10592=ORIENTED_EDGE('',*,*,#7700,.T.);
#10593=ORIENTED_EDGE('',*,*,#7701,.T.);
#10594=ORIENTED_EDGE('',*,*,#7697,.F.);
#10595=ORIENTED_EDGE('',*,*,#7578,.T.);
#10596=ORIENTED_EDGE('',*,*,#7702,.T.);
#10597=ORIENTED_EDGE('',*,*,#7703,.T.);
#10598=ORIENTED_EDGE('',*,*,#7700,.F.);
#10599=ORIENTED_EDGE('',*,*,#7584,.T.);
#10600=ORIENTED_EDGE('',*,*,#7704,.T.);
#10601=ORIENTED_EDGE('',*,*,#7705,.T.);
#10602=ORIENTED_EDGE('',*,*,#7702,.F.);
#10603=ORIENTED_EDGE('',*,*,#7706,.T.);
#10604=ORIENTED_EDGE('',*,*,#7707,.T.);
#10605=ORIENTED_EDGE('',*,*,#7708,.T.);
#10606=ORIENTED_EDGE('',*,*,#7704,.F.);
#10607=ORIENTED_EDGE('',*,*,#7610,.T.);
#10608=ORIENTED_EDGE('',*,*,#7709,.T.);
#10609=ORIENTED_EDGE('',*,*,#7710,.T.);
#10610=ORIENTED_EDGE('',*,*,#7707,.F.);
#10611=ORIENTED_EDGE('',*,*,#7615,.T.);
#10612=ORIENTED_EDGE('',*,*,#7711,.T.);
#10613=ORIENTED_EDGE('',*,*,#7712,.T.);
#10614=ORIENTED_EDGE('',*,*,#7709,.F.);
#10615=ORIENTED_EDGE('',*,*,#7621,.T.);
#10616=ORIENTED_EDGE('',*,*,#7699,.F.);
#10617=ORIENTED_EDGE('',*,*,#7713,.T.);
#10618=ORIENTED_EDGE('',*,*,#7711,.F.);
#10619=ORIENTED_EDGE('',*,*,#7714,.T.);
#10620=ORIENTED_EDGE('',*,*,#7706,.F.);
#10621=ORIENTED_EDGE('',*,*,#7583,.F.);
#10622=ORIENTED_EDGE('',*,*,#7715,.F.);
#10623=ORIENTED_EDGE('',*,*,#7611,.T.);
#10624=ORIENTED_EDGE('',*,*,#7698,.F.);
#10625=ORIENTED_EDGE('',*,*,#7701,.F.);
#10626=ORIENTED_EDGE('',*,*,#7703,.F.);
#10627=ORIENTED_EDGE('',*,*,#7705,.F.);
#10628=ORIENTED_EDGE('',*,*,#7708,.F.);
#10629=ORIENTED_EDGE('',*,*,#7710,.F.);
#10630=ORIENTED_EDGE('',*,*,#7712,.F.);
#10631=ORIENTED_EDGE('',*,*,#7713,.F.);
#10632=ORIENTED_EDGE('',*,*,#7716,.F.);
#10633=ORIENTED_EDGE('',*,*,#7717,.F.);
#10634=ORIENTED_EDGE('',*,*,#7718,.F.);
#10635=ORIENTED_EDGE('',*,*,#7719,.F.);
#10636=ORIENTED_EDGE('',*,*,#7720,.F.);
#10637=ORIENTED_EDGE('',*,*,#7721,.F.);
#10638=ORIENTED_EDGE('',*,*,#7722,.F.);
#10639=ORIENTED_EDGE('',*,*,#7723,.F.);
#10640=ORIENTED_EDGE('',*,*,#7724,.F.);
#10641=ORIENTED_EDGE('',*,*,#7725,.F.);
#10642=ORIENTED_EDGE('',*,*,#7726,.F.);
#10643=ORIENTED_EDGE('',*,*,#7727,.F.);
#10644=ORIENTED_EDGE('',*,*,#7728,.F.);
#10645=ORIENTED_EDGE('',*,*,#7729,.F.);
#10646=ORIENTED_EDGE('',*,*,#7730,.F.);
#10647=ORIENTED_EDGE('',*,*,#7731,.F.);
#10648=ORIENTED_EDGE('',*,*,#7732,.T.);
#10649=ORIENTED_EDGE('',*,*,#7733,.T.);
#10650=ORIENTED_EDGE('',*,*,#7656,.T.);
#10651=ORIENTED_EDGE('',*,*,#7691,.F.);
#10652=ORIENTED_EDGE('',*,*,#7734,.T.);
#10653=ORIENTED_EDGE('',*,*,#7735,.T.);
#10654=ORIENTED_EDGE('',*,*,#7733,.F.);
#10655=ORIENTED_EDGE('',*,*,#7736,.T.);
#10656=ORIENTED_EDGE('',*,*,#7737,.T.);
#10657=ORIENTED_EDGE('',*,*,#7738,.T.);
#10658=ORIENTED_EDGE('',*,*,#7734,.F.);
#10659=ORIENTED_EDGE('',*,*,#7739,.T.);
#10660=ORIENTED_EDGE('',*,*,#7740,.T.);
#10661=ORIENTED_EDGE('',*,*,#7688,.T.);
#10662=ORIENTED_EDGE('',*,*,#7737,.F.);
#10663=ORIENTED_EDGE('',*,*,#7741,.T.);
#10664=ORIENTED_EDGE('',*,*,#7639,.T.);
#10665=ORIENTED_EDGE('',*,*,#7740,.F.);
#10666=ORIENTED_EDGE('',*,*,#7742,.T.);
#10667=ORIENTED_EDGE('',*,*,#7695,.F.);
#10668=ORIENTED_EDGE('',*,*,#7742,.F.);
#10669=ORIENTED_EDGE('',*,*,#7741,.F.);
#10670=ORIENTED_EDGE('',*,*,#7739,.F.);
#10671=ORIENTED_EDGE('',*,*,#7736,.F.);
#10672=ORIENTED_EDGE('',*,*,#7732,.F.);
#10673=ORIENTED_EDGE('',*,*,#7694,.T.);
#10674=ORIENTED_EDGE('',*,*,#7743,.T.);
#10675=ORIENTED_EDGE('',*,*,#7744,.T.);
#10676=ORIENTED_EDGE('',*,*,#7641,.T.);
#10677=ORIENTED_EDGE('',*,*,#7696,.F.);
#10678=ORIENTED_EDGE('',*,*,#7745,.T.);
#10679=ORIENTED_EDGE('',*,*,#7675,.T.);
#10680=ORIENTED_EDGE('',*,*,#7744,.F.);
#10681=ORIENTED_EDGE('',*,*,#7746,.T.);
#10682=ORIENTED_EDGE('',*,*,#7747,.T.);
#10683=ORIENTED_EDGE('',*,*,#7674,.T.);
#10684=ORIENTED_EDGE('',*,*,#7745,.F.);
#10685=ORIENTED_EDGE('',*,*,#7748,.T.);
#10686=ORIENTED_EDGE('',*,*,#7749,.T.);
#10687=ORIENTED_EDGE('',*,*,#7672,.T.);
#10688=ORIENTED_EDGE('',*,*,#7747,.F.);
#10689=ORIENTED_EDGE('',*,*,#7750,.T.);
#10690=ORIENTED_EDGE('',*,*,#7654,.T.);
#10691=ORIENTED_EDGE('',*,*,#7749,.F.);
#10692=ORIENTED_EDGE('',*,*,#7751,.T.);
#10693=ORIENTED_EDGE('',*,*,#7689,.F.);
#10694=ORIENTED_EDGE('',*,*,#7751,.F.);
#10695=ORIENTED_EDGE('',*,*,#7750,.F.);
#10696=ORIENTED_EDGE('',*,*,#7748,.F.);
#10697=ORIENTED_EDGE('',*,*,#7746,.F.);
#10698=ORIENTED_EDGE('',*,*,#7743,.F.);
#10699=ORIENTED_EDGE('',*,*,#7692,.T.);
#10700=ORIENTED_EDGE('',*,*,#7718,.T.);
#10701=ORIENTED_EDGE('',*,*,#7752,.T.);
#10702=ORIENTED_EDGE('',*,*,#7753,.T.);
#10703=ORIENTED_EDGE('',*,*,#7754,.F.);
#10704=ORIENTED_EDGE('',*,*,#7716,.T.);
#10705=ORIENTED_EDGE('',*,*,#7755,.T.);
#10706=ORIENTED_EDGE('',*,*,#7756,.T.);
#10707=ORIENTED_EDGE('',*,*,#7757,.T.);
#10708=ORIENTED_EDGE('',*,*,#7758,.T.);
#10709=ORIENTED_EDGE('',*,*,#7755,.F.);
#10710=ORIENTED_EDGE('',*,*,#7719,.T.);
#10711=ORIENTED_EDGE('',*,*,#7754,.T.);
#10712=ORIENTED_EDGE('',*,*,#7717,.T.);
#10713=ORIENTED_EDGE('',*,*,#7757,.F.);
#10714=ORIENTED_EDGE('',*,*,#7759,.T.);
#10715=ORIENTED_EDGE('',*,*,#7752,.F.);
#10716=ORIENTED_EDGE('',*,*,#7759,.F.);
#10717=ORIENTED_EDGE('',*,*,#7760,.T.);
#10718=ORIENTED_EDGE('',*,*,#7761,.T.);
#10719=ORIENTED_EDGE('',*,*,#7762,.F.);
#10720=ORIENTED_EDGE('',*,*,#7756,.F.);
#10721=ORIENTED_EDGE('',*,*,#7763,.T.);
#10722=ORIENTED_EDGE('',*,*,#7764,.T.);
#10723=ORIENTED_EDGE('',*,*,#7760,.F.);
#10724=ORIENTED_EDGE('',*,*,#7765,.T.);
#10725=ORIENTED_EDGE('',*,*,#7730,.T.);
#10726=ORIENTED_EDGE('',*,*,#7766,.T.);
#10727=ORIENTED_EDGE('',*,*,#7767,.T.);
#10728=ORIENTED_EDGE('',*,*,#7768,.F.);
#10729=ORIENTED_EDGE('',*,*,#7728,.T.);
#10730=ORIENTED_EDGE('',*,*,#7769,.T.);
#10731=ORIENTED_EDGE('',*,*,#7770,.T.);
#10732=ORIENTED_EDGE('',*,*,#7771,.T.);
#10733=ORIENTED_EDGE('',*,*,#7772,.T.);
#10734=ORIENTED_EDGE('',*,*,#7769,.F.);
#10735=ORIENTED_EDGE('',*,*,#7731,.T.);
#10736=ORIENTED_EDGE('',*,*,#7768,.T.);
#10737=ORIENTED_EDGE('',*,*,#7729,.T.);
#10738=ORIENTED_EDGE('',*,*,#7771,.F.);
#10739=ORIENTED_EDGE('',*,*,#7773,.T.);
#10740=ORIENTED_EDGE('',*,*,#7766,.F.);
#10741=ORIENTED_EDGE('',*,*,#7773,.F.);
#10742=ORIENTED_EDGE('',*,*,#7774,.T.);
#10743=ORIENTED_EDGE('',*,*,#7775,.T.);
#10744=ORIENTED_EDGE('',*,*,#7776,.F.);
#10745=ORIENTED_EDGE('',*,*,#7770,.F.);
#10746=ORIENTED_EDGE('',*,*,#7777,.T.);
#10747=ORIENTED_EDGE('',*,*,#7778,.T.);
#10748=ORIENTED_EDGE('',*,*,#7774,.F.);
#10749=ORIENTED_EDGE('',*,*,#7779,.T.);
#10750=ORIENTED_EDGE('',*,*,#7722,.T.);
#10751=ORIENTED_EDGE('',*,*,#7780,.T.);
#10752=ORIENTED_EDGE('',*,*,#7781,.T.);
#10753=ORIENTED_EDGE('',*,*,#7782,.F.);
#10754=ORIENTED_EDGE('',*,*,#7720,.T.);
#10755=ORIENTED_EDGE('',*,*,#7783,.T.);
#10756=ORIENTED_EDGE('',*,*,#7784,.T.);
#10757=ORIENTED_EDGE('',*,*,#7785,.T.);
#10758=ORIENTED_EDGE('',*,*,#7786,.T.);
#10759=ORIENTED_EDGE('',*,*,#7783,.F.);
#10760=ORIENTED_EDGE('',*,*,#7723,.T.);
#10761=ORIENTED_EDGE('',*,*,#7782,.T.);
#10762=ORIENTED_EDGE('',*,*,#7721,.T.);
#10763=ORIENTED_EDGE('',*,*,#7785,.F.);
#10764=ORIENTED_EDGE('',*,*,#7787,.T.);
#10765=ORIENTED_EDGE('',*,*,#7780,.F.);
#10766=ORIENTED_EDGE('',*,*,#7787,.F.);
#10767=ORIENTED_EDGE('',*,*,#7788,.T.);
#10768=ORIENTED_EDGE('',*,*,#7789,.T.);
#10769=ORIENTED_EDGE('',*,*,#7790,.F.);
#10770=ORIENTED_EDGE('',*,*,#7784,.F.);
#10771=ORIENTED_EDGE('',*,*,#7791,.T.);
#10772=ORIENTED_EDGE('',*,*,#7792,.T.);
#10773=ORIENTED_EDGE('',*,*,#7788,.F.);
#10774=ORIENTED_EDGE('',*,*,#7793,.T.);
#10775=ORIENTED_EDGE('',*,*,#7726,.T.);
#10776=ORIENTED_EDGE('',*,*,#7794,.T.);
#10777=ORIENTED_EDGE('',*,*,#7795,.T.);
#10778=ORIENTED_EDGE('',*,*,#7796,.F.);
#10779=ORIENTED_EDGE('',*,*,#7724,.T.);
#10780=ORIENTED_EDGE('',*,*,#7797,.T.);
#10781=ORIENTED_EDGE('',*,*,#7798,.T.);
#10782=ORIENTED_EDGE('',*,*,#7799,.T.);
#10783=ORIENTED_EDGE('',*,*,#7800,.T.);
#10784=ORIENTED_EDGE('',*,*,#7797,.F.);
#10785=ORIENTED_EDGE('',*,*,#7727,.T.);
#10786=ORIENTED_EDGE('',*,*,#7796,.T.);
#10787=ORIENTED_EDGE('',*,*,#7725,.T.);
#10788=ORIENTED_EDGE('',*,*,#7799,.F.);
#10789=ORIENTED_EDGE('',*,*,#7801,.T.);
#10790=ORIENTED_EDGE('',*,*,#7794,.F.);
#10791=ORIENTED_EDGE('',*,*,#7801,.F.);
#10792=ORIENTED_EDGE('',*,*,#7802,.T.);
#10793=ORIENTED_EDGE('',*,*,#7803,.T.);
#10794=ORIENTED_EDGE('',*,*,#7804,.F.);
#10795=ORIENTED_EDGE('',*,*,#7798,.F.);
#10796=ORIENTED_EDGE('',*,*,#7805,.T.);
#10797=ORIENTED_EDGE('',*,*,#7806,.T.);
#10798=ORIENTED_EDGE('',*,*,#7802,.F.);
#10799=ORIENTED_EDGE('',*,*,#7807,.T.);
#10800=ORIENTED_EDGE('',*,*,#7579,.F.);
#10801=ORIENTED_EDGE('',*,*,#7808,.T.);
#10802=ORIENTED_EDGE('',*,*,#7809,.F.);
#10803=ORIENTED_EDGE('',*,*,#7808,.F.);
#10804=ORIENTED_EDGE('',*,*,#7793,.F.);
#10805=ORIENTED_EDGE('',*,*,#7810,.T.);
#10806=ORIENTED_EDGE('',*,*,#7811,.F.);
#10807=ORIENTED_EDGE('',*,*,#7810,.F.);
#10808=ORIENTED_EDGE('',*,*,#7807,.F.);
#10809=ORIENTED_EDGE('',*,*,#7812,.T.);
#10810=ORIENTED_EDGE('',*,*,#7813,.F.);
#10811=ORIENTED_EDGE('',*,*,#7812,.F.);
#10812=ORIENTED_EDGE('',*,*,#7765,.F.);
#10813=ORIENTED_EDGE('',*,*,#7814,.T.);
#10814=ORIENTED_EDGE('',*,*,#7815,.F.);
#10815=ORIENTED_EDGE('',*,*,#7814,.F.);
#10816=ORIENTED_EDGE('',*,*,#7779,.F.);
#10817=ORIENTED_EDGE('',*,*,#7816,.T.);
#10818=ORIENTED_EDGE('',*,*,#7616,.F.);
#10819=ORIENTED_EDGE('',*,*,#7816,.F.);
#10820=ORIENTED_EDGE('',*,*,#7800,.F.);
#10821=ORIENTED_EDGE('',*,*,#7817,.T.);
#10822=ORIENTED_EDGE('',*,*,#7818,.T.);
#10823=ORIENTED_EDGE('',*,*,#7805,.F.);
#10824=ORIENTED_EDGE('',*,*,#7795,.F.);
#10825=ORIENTED_EDGE('',*,*,#7804,.T.);
#10826=ORIENTED_EDGE('',*,*,#7819,.T.);
#10827=ORIENTED_EDGE('',*,*,#7817,.F.);
#10828=ORIENTED_EDGE('',*,*,#7815,.T.);
#10829=ORIENTED_EDGE('',*,*,#7803,.F.);
#10830=ORIENTED_EDGE('',*,*,#7806,.F.);
#10831=ORIENTED_EDGE('',*,*,#7818,.F.);
#10832=ORIENTED_EDGE('',*,*,#7819,.F.);
#10833=ORIENTED_EDGE('',*,*,#7786,.F.);
#10834=ORIENTED_EDGE('',*,*,#7820,.T.);
#10835=ORIENTED_EDGE('',*,*,#7821,.T.);
#10836=ORIENTED_EDGE('',*,*,#7791,.F.);
#10837=ORIENTED_EDGE('',*,*,#7781,.F.);
#10838=ORIENTED_EDGE('',*,*,#7790,.T.);
#10839=ORIENTED_EDGE('',*,*,#7822,.T.);
#10840=ORIENTED_EDGE('',*,*,#7820,.F.);
#10841=ORIENTED_EDGE('',*,*,#7813,.T.);
#10842=ORIENTED_EDGE('',*,*,#7789,.F.);
#10843=ORIENTED_EDGE('',*,*,#7792,.F.);
#10844=ORIENTED_EDGE('',*,*,#7821,.F.);
#10845=ORIENTED_EDGE('',*,*,#7822,.F.);
#10846=ORIENTED_EDGE('',*,*,#7772,.F.);
#10847=ORIENTED_EDGE('',*,*,#7823,.T.);
#10848=ORIENTED_EDGE('',*,*,#7824,.T.);
#10849=ORIENTED_EDGE('',*,*,#7777,.F.);
#10850=ORIENTED_EDGE('',*,*,#7767,.F.);
#10851=ORIENTED_EDGE('',*,*,#7776,.T.);
#10852=ORIENTED_EDGE('',*,*,#7825,.T.);
#10853=ORIENTED_EDGE('',*,*,#7823,.F.);
#10854=ORIENTED_EDGE('',*,*,#7811,.T.);
#10855=ORIENTED_EDGE('',*,*,#7775,.F.);
#10856=ORIENTED_EDGE('',*,*,#7778,.F.);
#10857=ORIENTED_EDGE('',*,*,#7824,.F.);
#10858=ORIENTED_EDGE('',*,*,#7825,.F.);
#10859=ORIENTED_EDGE('',*,*,#7758,.F.);
#10860=ORIENTED_EDGE('',*,*,#7826,.T.);
#10861=ORIENTED_EDGE('',*,*,#7827,.T.);
#10862=ORIENTED_EDGE('',*,*,#7763,.F.);
#10863=ORIENTED_EDGE('',*,*,#7753,.F.);
#10864=ORIENTED_EDGE('',*,*,#7762,.T.);
#10865=ORIENTED_EDGE('',*,*,#7828,.T.);
#10866=ORIENTED_EDGE('',*,*,#7826,.F.);
#10867=ORIENTED_EDGE('',*,*,#7809,.T.);
#10868=ORIENTED_EDGE('',*,*,#7761,.F.);
#10869=ORIENTED_EDGE('',*,*,#7764,.F.);
#10870=ORIENTED_EDGE('',*,*,#7827,.F.);
#10871=ORIENTED_EDGE('',*,*,#7828,.F.);
#10872=ORIENTED_EDGE('',*,*,#7686,.F.);
#10873=ORIENTED_EDGE('',*,*,#7829,.T.);
#10874=ORIENTED_EDGE('',*,*,#7738,.F.);
#10875=ORIENTED_EDGE('',*,*,#7687,.F.);
#10876=ORIENTED_EDGE('',*,*,#7685,.F.);
#10877=ORIENTED_EDGE('',*,*,#7657,.T.);
#10878=ORIENTED_EDGE('',*,*,#7735,.F.);
#10879=ORIENTED_EDGE('',*,*,#7829,.F.);
#10880=ORIENTED_EDGE('',*,*,#7597,.F.);
#10881=ORIENTED_EDGE('',*,*,#7606,.F.);
#10882=ORIENTED_EDGE('',*,*,#7651,.T.);
#10883=ORIENTED_EDGE('',*,*,#7601,.F.);
#10884=ORIENTED_EDGE('',*,*,#7604,.F.);
#10885=ORIENTED_EDGE('',*,*,#7569,.F.);
#10886=ORIENTED_EDGE('',*,*,#7644,.T.);
#10887=ORIENTED_EDGE('',*,*,#7564,.F.);
#10888=ORIENTED_EDGE('',*,*,#7567,.F.);
#10889=ORIENTED_EDGE('',*,*,#7714,.F.);
#10890=ORIENTED_EDGE('',*,*,#7620,.F.);
#10891=ORIENTED_EDGE('',*,*,#7830,.F.);
#10892=ORIENTED_EDGE('',*,*,#7574,.T.);
#10893=ORIENTED_EDGE('',*,*,#7670,.F.);
#10894=ORIENTED_EDGE('',*,*,#7612,.T.);
#10895=ORIENTED_EDGE('',*,*,#7715,.T.);
#10896=ORIENTED_EDGE('',*,*,#7582,.T.);
#10897=ORIENTED_EDGE('',*,*,#7660,.F.);
#10898=ORIENTED_EDGE('',*,*,#7662,.F.);
#10899=ORIENTED_EDGE('',*,*,#7665,.F.);
#10900=ORIENTED_EDGE('',*,*,#7668,.F.);
#10901=ORIENTED_EDGE('',*,*,#7634,.F.);
#10902=ORIENTED_EDGE('',*,*,#7575,.T.);
#10903=ORIENTED_EDGE('',*,*,#7830,.T.);
#10904=ORIENTED_EDGE('',*,*,#7619,.T.);
#10905=ORIENTED_EDGE('',*,*,#7624,.F.);
#10906=ORIENTED_EDGE('',*,*,#7626,.F.);
#10907=ORIENTED_EDGE('',*,*,#7629,.F.);
#10908=ORIENTED_EDGE('',*,*,#7632,.F.);
#12715=PLANE('',#14436);
#12716=PLANE('',#14444);
#12717=PLANE('',#14453);
#12718=PLANE('',#14463);
#12719=PLANE('',#14471);
#12720=PLANE('',#14477);
#12721=PLANE('',#14481);
#12722=PLANE('',#14485);
#12723=PLANE('',#14486);
#12724=PLANE('',#14489);
#12725=PLANE('',#14492);
#12726=PLANE('',#14493);
#12727=PLANE('',#14497);
#12728=PLANE('',#14501);
#12729=PLANE('',#14504);
#12730=PLANE('',#14509);
#12731=PLANE('',#14511);
#12732=PLANE('',#14513);
#12733=PLANE('',#14516);
#12734=PLANE('',#14519);
#12735=PLANE('',#14520);
#12736=PLANE('',#14521);
#12737=PLANE('',#14524);
#12738=PLANE('',#14527);
#12739=PLANE('',#14530);
#12740=PLANE('',#14533);
#12741=PLANE('',#14534);
#12742=PLANE('',#14535);
#12743=PLANE('',#14536);
#12744=PLANE('',#14540);
#12745=PLANE('',#14543);
#12746=PLANE('',#14544);
#12747=PLANE('',#14545);
#12748=PLANE('',#14548);
#12749=PLANE('',#14551);
#12750=PLANE('',#14552);
#12751=PLANE('',#14553);
#12752=PLANE('',#14554);
#12753=PLANE('',#14555);
#12754=PLANE('',#14556);
#12755=PLANE('',#14557);
#12756=PLANE('',#14558);
#12757=PLANE('',#14560);
#12758=PLANE('',#14561);
#12759=PLANE('',#14562);
#12760=PLANE('',#14563);
#12761=PLANE('',#14564);
#12762=PLANE('',#14565);
#12763=PLANE('',#14567);
#12764=PLANE('',#14568);
#12765=PLANE('',#14569);
#12766=PLANE('',#14570);
#12767=PLANE('',#14571);
#12768=PLANE('',#14572);
#12769=PLANE('',#14574);
#12770=PLANE('',#14575);
#12771=PLANE('',#14576);
#12772=PLANE('',#14577);
#12773=PLANE('',#14578);
#12774=PLANE('',#14579);
#12775=PLANE('',#14590);
#12776=PLANE('',#14591);
#12777=PLANE('',#14592);
#12778=PLANE('',#14593);
#12779=PLANE('',#14594);
#12780=PLANE('',#14595);
#12781=PLANE('',#14596);
#12782=PLANE('',#14597);
#12783=PLANE('',#14598);
#12784=PLANE('',#14599);
#12785=PLANE('',#14600);
#12786=PLANE('',#14601);
#12787=PLANE('',#14602);
#12788=PLANE('',#14604);
#12789=PLANE('',#14605);
#12790=PLANE('',#14606);
#12791=PLANE('',#14607);
#12792=PLANE('',#14608);
#12793=PLANE('',#14609);
#13358=ADVANCED_FACE('',(#1595),#1181,.T.);
#13359=ADVANCED_FACE('',(#1596),#12715,.T.);
#13360=ADVANCED_FACE('',(#1597),#1182,.T.);
#13361=ADVANCED_FACE('',(#1598),#726,.T.);
#13362=ADVANCED_FACE('',(#1599,#627),#12716,.T.);
#13363=ADVANCED_FACE('',(#1600),#727,.T.);
#13364=ADVANCED_FACE('',(#1601),#1183,.F.);
#13365=ADVANCED_FACE('',(#1602,#628),#12717,.T.);
#13366=ADVANCED_FACE('',(#1603),#728,.F.);
#13367=ADVANCED_FACE('',(#1604),#1184,.T.);
#13368=ADVANCED_FACE('',(#1605),#12718,.T.);
#13369=ADVANCED_FACE('',(#1606),#1185,.T.);
#13370=ADVANCED_FACE('',(#1607),#729,.T.);
#13371=ADVANCED_FACE('',(#1608,#629),#12719,.T.);
#13372=ADVANCED_FACE('',(#1609),#730,.T.);
#13373=ADVANCED_FACE('',(#1610),#12720,.T.);
#13374=ADVANCED_FACE('',(#1611),#1186,.T.);
#13375=ADVANCED_FACE('',(#1612),#12721,.T.);
#13376=ADVANCED_FACE('',(#1613),#1187,.T.);
#13377=ADVANCED_FACE('',(#1614),#12722,.T.);
#13378=ADVANCED_FACE('',(#1615),#12723,.T.);
#13379=ADVANCED_FACE('',(#1616),#731,.T.);
#13380=ADVANCED_FACE('',(#1617),#12724,.T.);
#13381=ADVANCED_FACE('',(#1618),#732,.T.);
#13382=ADVANCED_FACE('',(#1619),#12725,.T.);
#13383=ADVANCED_FACE('',(#1620),#12726,.T.);
#13384=ADVANCED_FACE('',(#1621),#1188,.T.);
#13385=ADVANCED_FACE('',(#1622),#12727,.T.);
#13386=ADVANCED_FACE('',(#1623),#1189,.T.);
#13387=ADVANCED_FACE('',(#1624),#12728,.T.);
#13388=ADVANCED_FACE('',(#1625),#733,.T.);
#13389=ADVANCED_FACE('',(#1626),#12729,.T.);
#13390=ADVANCED_FACE('',(#1627),#734,.T.);
#13391=ADVANCED_FACE('',(#1628),#1190,.T.);
#13392=ADVANCED_FACE('',(#1629),#12730,.T.);
#13393=ADVANCED_FACE('',(#1630),#1191,.T.);
#13394=ADVANCED_FACE('',(#1631),#12731,.T.);
#13395=ADVANCED_FACE('',(#1632),#1192,.T.);
#13396=ADVANCED_FACE('',(#1633),#12732,.T.);
#13397=ADVANCED_FACE('',(#1634),#1193,.T.);
#13398=ADVANCED_FACE('',(#1635),#12733,.T.);
#13399=ADVANCED_FACE('',(#1636),#735,.T.);
#13400=ADVANCED_FACE('',(#1637),#12734,.T.);
#13401=ADVANCED_FACE('',(#1638),#12735,.F.);
#13402=ADVANCED_FACE('',(#1639),#12736,.T.);
#13403=ADVANCED_FACE('',(#1640),#1194,.T.);
#13404=ADVANCED_FACE('',(#1641),#12737,.T.);
#13405=ADVANCED_FACE('',(#1642),#1195,.T.);
#13406=ADVANCED_FACE('',(#1643),#12738,.T.);
#13407=ADVANCED_FACE('',(#1644),#1196,.T.);
#13408=ADVANCED_FACE('',(#1645),#12739,.T.);
#13409=ADVANCED_FACE('',(#1646),#1197,.T.);
#13410=ADVANCED_FACE('',(#1647),#12740,.T.);
#13411=ADVANCED_FACE('',(#1648),#12741,.T.);
#13412=ADVANCED_FACE('',(#1649,#630,#631,#632,#633),#12742,.F.);
#13413=ADVANCED_FACE('',(#1650),#12743,.T.);
#13414=ADVANCED_FACE('',(#1651),#1198,.T.);
#13415=ADVANCED_FACE('',(#1652),#12744,.T.);
#13416=ADVANCED_FACE('',(#1653),#1199,.T.);
#13417=ADVANCED_FACE('',(#1654),#12745,.T.);
#13418=ADVANCED_FACE('',(#1655),#12746,.F.);
#13419=ADVANCED_FACE('',(#1656),#12747,.T.);
#13420=ADVANCED_FACE('',(#1657),#1200,.T.);
#13421=ADVANCED_FACE('',(#1658),#12748,.T.);
#13422=ADVANCED_FACE('',(#1659),#1201,.T.);
#13423=ADVANCED_FACE('',(#1660),#12749,.T.);
#13424=ADVANCED_FACE('',(#1661),#12750,.F.);
#13425=ADVANCED_FACE('',(#1662),#12751,.T.);
#13426=ADVANCED_FACE('',(#1663),#12752,.T.);
#13427=ADVANCED_FACE('',(#1664),#12753,.T.);
#13428=ADVANCED_FACE('',(#1665),#12754,.T.);
#13429=ADVANCED_FACE('',(#1666),#12755,.F.);
#13430=ADVANCED_FACE('',(#1667,#634),#12756,.F.);
#13431=ADVANCED_FACE('',(#1668),#12757,.T.);
#13432=ADVANCED_FACE('',(#1669),#12758,.T.);
#13433=ADVANCED_FACE('',(#1670),#12759,.T.);
#13434=ADVANCED_FACE('',(#1671),#12760,.T.);
#13435=ADVANCED_FACE('',(#1672),#12761,.F.);
#13436=ADVANCED_FACE('',(#1673,#635),#12762,.F.);
#13437=ADVANCED_FACE('',(#1674),#12763,.T.);
#13438=ADVANCED_FACE('',(#1675),#12764,.T.);
#13439=ADVANCED_FACE('',(#1676),#12765,.T.);
#13440=ADVANCED_FACE('',(#1677),#12766,.T.);
#13441=ADVANCED_FACE('',(#1678),#12767,.F.);
#13442=ADVANCED_FACE('',(#1679,#636),#12768,.F.);
#13443=ADVANCED_FACE('',(#1680),#12769,.T.);
#13444=ADVANCED_FACE('',(#1681),#12770,.T.);
#13445=ADVANCED_FACE('',(#1682),#12771,.T.);
#13446=ADVANCED_FACE('',(#1683),#12772,.T.);
#13447=ADVANCED_FACE('',(#1684),#12773,.F.);
#13448=ADVANCED_FACE('',(#1685,#637),#12774,.F.);
#13449=ADVANCED_FACE('',(#1686),#736,.F.);
#13450=ADVANCED_FACE('',(#1687),#737,.F.);
#13451=ADVANCED_FACE('',(#1688),#738,.F.);
#13452=ADVANCED_FACE('',(#1689),#739,.F.);
#13453=ADVANCED_FACE('',(#1690),#740,.F.);
#13454=ADVANCED_FACE('',(#1691),#12775,.F.);
#13455=ADVANCED_FACE('',(#1692,#638),#12776,.F.);
#13456=ADVANCED_FACE('',(#1693),#12777,.F.);
#13457=ADVANCED_FACE('',(#1694),#12778,.F.);
#13458=ADVANCED_FACE('',(#1695,#639),#12779,.F.);
#13459=ADVANCED_FACE('',(#1696),#12780,.F.);
#13460=ADVANCED_FACE('',(#1697),#12781,.F.);
#13461=ADVANCED_FACE('',(#1698,#640),#12782,.F.);
#13462=ADVANCED_FACE('',(#1699),#12783,.F.);
#13463=ADVANCED_FACE('',(#1700),#12784,.F.);
#13464=ADVANCED_FACE('',(#1701,#641),#12785,.F.);
#13465=ADVANCED_FACE('',(#1702),#12786,.F.);
#13466=ADVANCED_FACE('',(#1703),#12787,.T.);
#13467=ADVANCED_FACE('',(#1704),#741,.T.);
#13468=ADVANCED_FACE('',(#1705),#12788,.T.);
#13469=ADVANCED_FACE('',(#1706),#12789,.T.);
#13470=ADVANCED_FACE('',(#1707),#12790,.T.);
#13471=ADVANCED_FACE('',(#1708),#12791,.T.);
#13472=ADVANCED_FACE('',(#1709),#12792,.F.);
#13473=ADVANCED_FACE('',(#1710),#12793,.F.);
#13811=CLOSED_SHELL('',(#13358,#13359,#13360,#13361,#13362,#13363,#13364,
#13365,#13366,#13367,#13368,#13369,#13370,#13371,#13372,#13373,#13374,#13375,
#13376,#13377,#13378,#13379,#13380,#13381,#13382,#13383,#13384,#13385,#13386,
#13387,#13388,#13389,#13390,#13391,#13392,#13393,#13394,#13395,#13396,#13397,
#13398,#13399,#13400,#13401,#13402,#13403,#13404,#13405,#13406,#13407,#13408,
#13409,#13410,#13411,#13412,#13413,#13414,#13415,#13416,#13417,#13418,#13419,
#13420,#13421,#13422,#13423,#13424,#13425,#13426,#13427,#13428,#13429,#13430,
#13431,#13432,#13433,#13434,#13435,#13436,#13437,#13438,#13439,#13440,#13441,
#13442,#13443,#13444,#13445,#13446,#13447,#13448,#13449,#13450,#13451,#13452,
#13453,#13454,#13455,#13456,#13457,#13458,#13459,#13460,#13461,#13462,#13463,
#13464,#13465,#13466,#13467,#13468,#13469,#13470,#13471,#13472,#13473));
#14432=AXIS2_PLACEMENT_3D('',#25937,#16381,#16382);
#14433=AXIS2_PLACEMENT_3D('',#25938,#16383,#16384);
#14434=AXIS2_PLACEMENT_3D('',#25945,#16385,#16386);
#14435=AXIS2_PLACEMENT_3D('',#25948,#16388,#16389);
#14436=AXIS2_PLACEMENT_3D('',#25949,#16390,#16391);
#14437=AXIS2_PLACEMENT_3D('',#25955,#16395,#16396);
#14438=AXIS2_PLACEMENT_3D('',#25961,#16397,#16398);
#14439=AXIS2_PLACEMENT_3D('',#25962,#16399,#16400);
#14440=AXIS2_PLACEMENT_3D('',#25963,#16401,#16402);
#14441=AXIS2_PLACEMENT_3D('',#25969,#16405,#16406);
#14442=AXIS2_PLACEMENT_3D('',#25973,#16408,#16409);
#14443=AXIS2_PLACEMENT_3D('',#25974,#16410,#16411);
#14444=AXIS2_PLACEMENT_3D('',#25975,#16412,#16413);
#14445=AXIS2_PLACEMENT_3D('',#25980,#16416,#16417);
#14446=AXIS2_PLACEMENT_3D('',#25981,#16418,#16419);
#14447=AXIS2_PLACEMENT_3D('',#25985,#16421,#16422);
#14448=AXIS2_PLACEMENT_3D('',#25987,#16423,#16424);
#14449=AXIS2_PLACEMENT_3D('',#25990,#16426,#16427);
#14450=AXIS2_PLACEMENT_3D('',#25991,#16428,#16429);
#14451=AXIS2_PLACEMENT_3D('',#25993,#16430,#16431);
#14452=AXIS2_PLACEMENT_3D('',#25996,#16433,#16434);
#14453=AXIS2_PLACEMENT_3D('',#25997,#16435,#16436);
#14454=AXIS2_PLACEMENT_3D('',#26000,#16437,#16438);
#14455=AXIS2_PLACEMENT_3D('',#26004,#16440,#16441);
#14456=AXIS2_PLACEMENT_3D('',#26008,#16443,#16444);
#14457=AXIS2_PLACEMENT_3D('',#26012,#16446,#16447);
#14458=AXIS2_PLACEMENT_3D('',#26014,#16449,#16450);
#14459=AXIS2_PLACEMENT_3D('',#26017,#16452,#16453);
#14460=AXIS2_PLACEMENT_3D('',#26018,#16454,#16455);
#14461=AXIS2_PLACEMENT_3D('',#26025,#16456,#16457);
#14462=AXIS2_PLACEMENT_3D('',#26028,#16459,#16460);
#14463=AXIS2_PLACEMENT_3D('',#26029,#16461,#16462);
#14464=AXIS2_PLACEMENT_3D('',#26035,#16466,#16467);
#14465=AXIS2_PLACEMENT_3D('',#26041,#16468,#16469);
#14466=AXIS2_PLACEMENT_3D('',#26042,#16470,#16471);
#14467=AXIS2_PLACEMENT_3D('',#26043,#16472,#16473);
#14468=AXIS2_PLACEMENT_3D('',#26049,#16476,#16477);
#14469=AXIS2_PLACEMENT_3D('',#26053,#16479,#16480);
#14470=AXIS2_PLACEMENT_3D('',#26054,#16481,#16482);
#14471=AXIS2_PLACEMENT_3D('',#26055,#16483,#16484);
#14472=AXIS2_PLACEMENT_3D('',#26060,#16487,#16488);
#14473=AXIS2_PLACEMENT_3D('',#26061,#16489,#16490);
#14474=AXIS2_PLACEMENT_3D('',#26065,#16492,#16493);
#14475=AXIS2_PLACEMENT_3D('',#26067,#16494,#16495);
#14476=AXIS2_PLACEMENT_3D('',#26070,#16497,#16498);
#14477=AXIS2_PLACEMENT_3D('',#26071,#16499,#16500);
#14478=AXIS2_PLACEMENT_3D('',#26077,#16504,#16505);
#14479=AXIS2_PLACEMENT_3D('',#26081,#16507,#16508);
#14480=AXIS2_PLACEMENT_3D('',#26082,#16509,#16510);
#14481=AXIS2_PLACEMENT_3D('',#26083,#16511,#16512);
#14482=AXIS2_PLACEMENT_3D('',#26089,#16516,#16517);
#14483=AXIS2_PLACEMENT_3D('',#26093,#16519,#16520);
#14484=AXIS2_PLACEMENT_3D('',#26094,#16521,#16522);
#14485=AXIS2_PLACEMENT_3D('',#26095,#16523,#16524);
#14486=AXIS2_PLACEMENT_3D('',#26098,#16527,#16528);
#14487=AXIS2_PLACEMENT_3D('',#26115,#16538,#16539);
#14488=AXIS2_PLACEMENT_3D('',#26118,#16541,#16542);
#14489=AXIS2_PLACEMENT_3D('',#26119,#16543,#16544);
#14490=AXIS2_PLACEMENT_3D('',#26123,#16547,#16548);
#14491=AXIS2_PLACEMENT_3D('',#26126,#16550,#16551);
#14492=AXIS2_PLACEMENT_3D('',#26127,#16552,#16553);
#14493=AXIS2_PLACEMENT_3D('',#26142,#16562,#16563);
#14494=AXIS2_PLACEMENT_3D('',#26146,#16566,#16567);
#14495=AXIS2_PLACEMENT_3D('',#26150,#16569,#16570);
#14496=AXIS2_PLACEMENT_3D('',#26151,#16571,#16572);
#14497=AXIS2_PLACEMENT_3D('',#26152,#16573,#16574);
#14498=AXIS2_PLACEMENT_3D('',#26158,#16578,#16579);
#14499=AXIS2_PLACEMENT_3D('',#26161,#16581,#16582);
#14500=AXIS2_PLACEMENT_3D('',#26162,#16583,#16584);
#14501=AXIS2_PLACEMENT_3D('',#26163,#16585,#16586);
#14502=AXIS2_PLACEMENT_3D('',#26165,#16588,#16589);
#14503=AXIS2_PLACEMENT_3D('',#26168,#16591,#16592);
#14504=AXIS2_PLACEMENT_3D('',#26169,#16593,#16594);
#14505=AXIS2_PLACEMENT_3D('',#26173,#16597,#16598);
#14506=AXIS2_PLACEMENT_3D('',#26174,#16599,#16600);
#14507=AXIS2_PLACEMENT_3D('',#26175,#16601,#16602);
#14508=AXIS2_PLACEMENT_3D('',#26179,#16605,#16606);
#14509=AXIS2_PLACEMENT_3D('',#26180,#16607,#16608);
#14510=AXIS2_PLACEMENT_3D('',#26182,#16610,#16611);
#14511=AXIS2_PLACEMENT_3D('',#26184,#16613,#16614);
#14512=AXIS2_PLACEMENT_3D('',#26186,#16616,#16617);
#14513=AXIS2_PLACEMENT_3D('',#26188,#16619,#16620);
#14514=AXIS2_PLACEMENT_3D('',#26190,#16622,#16623);
#14515=AXIS2_PLACEMENT_3D('',#26193,#16625,#16626);
#14516=AXIS2_PLACEMENT_3D('',#26194,#16627,#16628);
#14517=AXIS2_PLACEMENT_3D('',#26196,#16630,#16631);
#14518=AXIS2_PLACEMENT_3D('',#26199,#16633,#16634);
#14519=AXIS2_PLACEMENT_3D('',#26200,#16635,#16636);
#14520=AXIS2_PLACEMENT_3D('',#26206,#16640,#16641);
#14521=AXIS2_PLACEMENT_3D('',#26212,#16645,#16646);
#14522=AXIS2_PLACEMENT_3D('',#26215,#16649,#16650);
#14523=AXIS2_PLACEMENT_3D('',#26219,#16652,#16653);
#14524=AXIS2_PLACEMENT_3D('',#26221,#16655,#16656);
#14525=AXIS2_PLACEMENT_3D('',#26225,#16659,#16660);
#14526=AXIS2_PLACEMENT_3D('',#26228,#16662,#16663);
#14527=AXIS2_PLACEMENT_3D('',#26229,#16664,#16665);
#14528=AXIS2_PLACEMENT_3D('',#26234,#16669,#16670);
#14529=AXIS2_PLACEMENT_3D('',#26237,#16672,#16673);
#14530=AXIS2_PLACEMENT_3D('',#26238,#16674,#16675);
#14531=AXIS2_PLACEMENT_3D('',#26242,#16678,#16679);
#14532=AXIS2_PLACEMENT_3D('',#26245,#16681,#16682);
#14533=AXIS2_PLACEMENT_3D('',#26246,#16683,#16684);
#14534=AXIS2_PLACEMENT_3D('',#26249,#16687,#16688);
#14535=AXIS2_PLACEMENT_3D('',#26251,#16690,#16691);
#14536=AXIS2_PLACEMENT_3D('',#26284,#16708,#16709);
#14537=AXIS2_PLACEMENT_3D('',#26288,#16712,#16713);
#14538=AXIS2_PLACEMENT_3D('',#26292,#16715,#16716);
#14539=AXIS2_PLACEMENT_3D('',#26293,#16717,#16718);
#14540=AXIS2_PLACEMENT_3D('',#26294,#16719,#16720);
#14541=AXIS2_PLACEMENT_3D('',#26299,#16724,#16725);
#14542=AXIS2_PLACEMENT_3D('',#26302,#16727,#16728);
#14543=AXIS2_PLACEMENT_3D('',#26303,#16729,#16730);
#14544=AXIS2_PLACEMENT_3D('',#26305,#16732,#16733);
#14545=AXIS2_PLACEMENT_3D('',#26306,#16734,#16735);
#14546=AXIS2_PLACEMENT_3D('',#26310,#16738,#16739);
#14547=AXIS2_PLACEMENT_3D('',#26313,#16741,#16742);
#14548=AXIS2_PLACEMENT_3D('',#26314,#16743,#16744);
#14549=AXIS2_PLACEMENT_3D('',#26318,#16747,#16748);
#14550=AXIS2_PLACEMENT_3D('',#26321,#16750,#16751);
#14551=AXIS2_PLACEMENT_3D('',#26322,#16752,#16753);
#14552=AXIS2_PLACEMENT_3D('',#26324,#16755,#16756);
#14553=AXIS2_PLACEMENT_3D('',#26325,#16757,#16758);
#14554=AXIS2_PLACEMENT_3D('',#26331,#16762,#16763);
#14555=AXIS2_PLACEMENT_3D('',#26337,#16767,#16768);
#14556=AXIS2_PLACEMENT_3D('',#26339,#16770,#16771);
#14557=AXIS2_PLACEMENT_3D('',#26341,#16773,#16774);
#14558=AXIS2_PLACEMENT_3D('',#26347,#16778,#16779);
#14559=AXIS2_PLACEMENT_3D('',#26352,#16782,#16783);
#14560=AXIS2_PLACEMENT_3D('',#26353,#16784,#16785);
#14561=AXIS2_PLACEMENT_3D('',#26359,#16789,#16790);
#14562=AXIS2_PLACEMENT_3D('',#26365,#16794,#16795);
#14563=AXIS2_PLACEMENT_3D('',#26367,#16797,#16798);
#14564=AXIS2_PLACEMENT_3D('',#26369,#16800,#16801);
#14565=AXIS2_PLACEMENT_3D('',#26375,#16805,#16806);
#14566=AXIS2_PLACEMENT_3D('',#26380,#16809,#16810);
#14567=AXIS2_PLACEMENT_3D('',#26381,#16811,#16812);
#14568=AXIS2_PLACEMENT_3D('',#26387,#16816,#16817);
#14569=AXIS2_PLACEMENT_3D('',#26393,#16821,#16822);
#14570=AXIS2_PLACEMENT_3D('',#26395,#16824,#16825);
#14571=AXIS2_PLACEMENT_3D('',#26397,#16827,#16828);
#14572=AXIS2_PLACEMENT_3D('',#26403,#16832,#16833);
#14573=AXIS2_PLACEMENT_3D('',#26408,#16836,#16837);
#14574=AXIS2_PLACEMENT_3D('',#26409,#16838,#16839);
#14575=AXIS2_PLACEMENT_3D('',#26415,#16843,#16844);
#14576=AXIS2_PLACEMENT_3D('',#26421,#16848,#16849);
#14577=AXIS2_PLACEMENT_3D('',#26423,#16851,#16852);
#14578=AXIS2_PLACEMENT_3D('',#26425,#16854,#16855);
#14579=AXIS2_PLACEMENT_3D('',#26431,#16859,#16860);
#14580=AXIS2_PLACEMENT_3D('',#26436,#16863,#16864);
#14581=AXIS2_PLACEMENT_3D('',#26437,#16865,#16866);
#14582=AXIS2_PLACEMENT_3D('',#26440,#16868,#16869);
#14583=AXIS2_PLACEMENT_3D('',#26441,#16870,#16871);
#14584=AXIS2_PLACEMENT_3D('',#26444,#16873,#16874);
#14585=AXIS2_PLACEMENT_3D('',#26445,#16875,#16876);
#14586=AXIS2_PLACEMENT_3D('',#26448,#16878,#16879);
#14587=AXIS2_PLACEMENT_3D('',#26449,#16880,#16881);
#14588=AXIS2_PLACEMENT_3D('',#26452,#16883,#16884);
#14589=AXIS2_PLACEMENT_3D('',#26453,#16885,#16886);
#14590=AXIS2_PLACEMENT_3D('',#26455,#16888,#16889);
#14591=AXIS2_PLACEMENT_3D('',#26459,#16892,#16893);
#14592=AXIS2_PLACEMENT_3D('',#26461,#16895,#16896);
#14593=AXIS2_PLACEMENT_3D('',#26462,#16897,#16898);
#14594=AXIS2_PLACEMENT_3D('',#26466,#16901,#16902);
#14595=AXIS2_PLACEMENT_3D('',#26468,#16904,#16905);
#14596=AXIS2_PLACEMENT_3D('',#26469,#16906,#16907);
#14597=AXIS2_PLACEMENT_3D('',#26473,#16910,#16911);
#14598=AXIS2_PLACEMENT_3D('',#26475,#16913,#16914);
#14599=AXIS2_PLACEMENT_3D('',#26476,#16915,#16916);
#14600=AXIS2_PLACEMENT_3D('',#26480,#16919,#16920);
#14601=AXIS2_PLACEMENT_3D('',#26482,#16922,#16923);
#14602=AXIS2_PLACEMENT_3D('',#26483,#16924,#16925);
#14603=AXIS2_PLACEMENT_3D('',#26485,#16927,#16928);
#14604=AXIS2_PLACEMENT_3D('',#26486,#16929,#16930);
#14605=AXIS2_PLACEMENT_3D('',#26487,#16931,#16932);
#14606=AXIS2_PLACEMENT_3D('',#26488,#16933,#16934);
#14607=AXIS2_PLACEMENT_3D('',#26489,#16935,#16936);
#14608=AXIS2_PLACEMENT_3D('',#26491,#16938,#16939);
#14609=AXIS2_PLACEMENT_3D('',#26492,#16940,#16941);
#16381=DIRECTION('axis',(0.,0.,1.));
#16382=DIRECTION('refdir',(1.,0.,0.));
#16383=DIRECTION('center_axis',(0.,-1.,0.));
#16384=DIRECTION('ref_axis',(-4.93432455388959E-16,0.,1.));
#16385=DIRECTION('center_axis',(0.,1.,0.));
#16386=DIRECTION('ref_axis',(-4.93432455388959E-16,0.,1.));
#16387=DIRECTION('',(-0.707106781186548,0.707106781186548,0.));
#16388=DIRECTION('center_axis',(0.,-1.,0.));
#16389=DIRECTION('ref_axis',(-4.93432455388959E-16,0.,1.));
#16390=DIRECTION('center_axis',(0.707106781186548,0.707106781186548,0.));
#16391=DIRECTION('ref_axis',(0.,0.,-1.));
#16392=DIRECTION('',(0.,0.,-1.));
#16393=DIRECTION('',(-0.707106781186548,0.707106781186548,0.));
#16394=DIRECTION('',(0.,0.,1.));
#16395=DIRECTION('center_axis',(0.,-1.,0.));
#16396=DIRECTION('ref_axis',(1.,0.,2.46716227694479E-16));
#16397=DIRECTION('center_axis',(0.,-1.,0.));
#16398=DIRECTION('ref_axis',(1.,0.,2.46716227694479E-16));
#16399=DIRECTION('center_axis',(0.,1.,0.));
#16400=DIRECTION('ref_axis',(1.,0.,2.46716227694479E-16));
#16401=DIRECTION('center_axis',(0.,-1.,0.));
#16402=DIRECTION('ref_axis',(1.,0.,2.46716227694479E-16));
#16403=DIRECTION('',(0.,-1.,0.));
#16404=DIRECTION('',(0.,-1.,0.));
#16405=DIRECTION('center_axis',(0.,-1.,0.));
#16406=DIRECTION('ref_axis',(1.,0.,2.46716227694479E-16));
#16407=DIRECTION('',(0.,-1.,0.));
#16408=DIRECTION('center_axis',(0.,1.,0.));
#16409=DIRECTION('ref_axis',(1.,0.,2.46716227694479E-16));
#16410=DIRECTION('center_axis',(0.707106781186548,-0.707106781186548,0.));
#16411=DIRECTION('ref_axis',(0.707106781186547,0.707106781186547,1.74454717631531E-16));
#16412=DIRECTION('center_axis',(1.,0.,0.));
#16413=DIRECTION('ref_axis',(0.,0.,1.));
#16414=DIRECTION('',(0.,-1.,0.));
#16415=DIRECTION('',(0.,0.,1.));
#16416=DIRECTION('center_axis',(-1.,0.,0.));
#16417=DIRECTION('ref_axis',(0.,0.,-1.));
#16418=DIRECTION('center_axis',(0.,-1.,0.));
#16419=DIRECTION('ref_axis',(-4.93432455388959E-16,0.,1.));
#16420=DIRECTION('',(0.,1.,0.));
#16421=DIRECTION('center_axis',(0.707106781186548,-0.707106781186548,0.));
#16422=DIRECTION('ref_axis',(-0.707106781186547,-0.707106781186547,-3.48909435263061E-16));
#16423=DIRECTION('center_axis',(0.,1.,0.));
#16424=DIRECTION('ref_axis',(-4.93432455388959E-16,0.,1.));
#16425=DIRECTION('',(0.,-1.,0.));
#16426=DIRECTION('center_axis',(0.,-1.,0.));
#16427=DIRECTION('ref_axis',(-4.93432455388959E-16,0.,1.));
#16428=DIRECTION('center_axis',(0.,1.,0.));
#16429=DIRECTION('ref_axis',(1.,0.,0.));
#16430=DIRECTION('center_axis',(0.,1.,0.));
#16431=DIRECTION('ref_axis',(1.,0.,0.));
#16432=DIRECTION('',(0.707106781186546,-0.707106781186549,-8.65956056235492E-17));
#16433=DIRECTION('center_axis',(0.,-1.,0.));
#16434=DIRECTION('ref_axis',(1.,0.,0.));
#16435=DIRECTION('center_axis',(0.,1.,0.));
#16436=DIRECTION('ref_axis',(1.,0.,0.));
#16437=DIRECTION('center_axis',(0.,-1.,0.));
#16438=DIRECTION('ref_axis',(2.22044604925031E-15,0.,1.));
#16439=DIRECTION('',(0.,0.,1.));
#16440=DIRECTION('center_axis',(0.,-1.,0.));
#16441=DIRECTION('ref_axis',(1.,0.,0.));
#16442=DIRECTION('',(1.,0.,0.));
#16443=DIRECTION('center_axis',(0.,-1.,0.));
#16444=DIRECTION('ref_axis',(-4.16333634234433E-16,0.,-1.));
#16445=DIRECTION('',(0.,0.,-1.));
#16446=DIRECTION('center_axis',(0.,-1.,0.));
#16447=DIRECTION('ref_axis',(-1.,0.,1.11022302462516E-15));
#16448=DIRECTION('',(-1.,0.,0.));
#16449=DIRECTION('center_axis',(0.,-1.,0.));
#16450=DIRECTION('ref_axis',(1.,0.,0.));
#16451=DIRECTION('',(0.,-1.,0.));
#16452=DIRECTION('center_axis',(0.,-1.,0.));
#16453=DIRECTION('ref_axis',(1.,0.,0.));
#16454=DIRECTION('center_axis',(0.,-1.,0.));
#16455=DIRECTION('ref_axis',(-1.85037170770859E-16,0.,-1.));
#16456=DIRECTION('center_axis',(0.,1.,0.));
#16457=DIRECTION('ref_axis',(-1.85037170770859E-16,0.,-1.));
#16458=DIRECTION('',(0.707106781186548,0.707106781186547,7.85046229341889E-16));
#16459=DIRECTION('center_axis',(0.,-1.,0.));
#16460=DIRECTION('ref_axis',(-1.85037170770859E-16,0.,-1.));
#16461=DIRECTION('center_axis',(-0.707106781186545,0.70710678118655,0.));
#16462=DIRECTION('ref_axis',(0.,0.,1.));
#16463=DIRECTION('',(0.,0.,1.));
#16464=DIRECTION('',(0.70710678118655,0.707106781186545,0.));
#16465=DIRECTION('',(0.,0.,-1.));
#16466=DIRECTION('center_axis',(0.,-1.,0.));
#16467=DIRECTION('ref_axis',(-1.,0.,0.));
#16468=DIRECTION('center_axis',(0.,-1.,0.));
#16469=DIRECTION('ref_axis',(-1.,0.,0.));
#16470=DIRECTION('center_axis',(0.,1.,0.));
#16471=DIRECTION('ref_axis',(-1.,0.,0.));
#16472=DIRECTION('center_axis',(0.,-1.,0.));
#16473=DIRECTION('ref_axis',(-1.,0.,0.));
#16474=DIRECTION('',(0.,-1.,0.));
#16475=DIRECTION('',(0.,-1.,0.));
#16476=DIRECTION('center_axis',(0.,-1.,0.));
#16477=DIRECTION('ref_axis',(-1.,0.,0.));
#16478=DIRECTION('',(0.,-1.,0.));
#16479=DIRECTION('center_axis',(0.,1.,0.));
#16480=DIRECTION('ref_axis',(-1.,0.,0.));
#16481=DIRECTION('center_axis',(-0.707106781186546,-0.707106781186549,0.));
#16482=DIRECTION('ref_axis',(-0.707106781186549,0.707106781186546,0.));
#16483=DIRECTION('center_axis',(-1.,0.,0.));
#16484=DIRECTION('ref_axis',(0.,0.,-1.));
#16485=DIRECTION('',(0.,-1.,0.));
#16486=DIRECTION('',(0.,0.,-1.));
#16487=DIRECTION('center_axis',(1.,0.,0.));
#16488=DIRECTION('ref_axis',(0.,0.,-1.));
#16489=DIRECTION('center_axis',(0.,-1.,0.));
#16490=DIRECTION('ref_axis',(-1.85037170770859E-16,0.,-1.));
#16491=DIRECTION('',(0.,1.,0.));
#16492=DIRECTION('center_axis',(-0.707106781186546,-0.707106781186549,0.));
#16493=DIRECTION('ref_axis',(0.707106781186549,-0.707106781186546,-1.30841038223648E-16));
#16494=DIRECTION('center_axis',(0.,1.,0.));
#16495=DIRECTION('ref_axis',(-1.85037170770859E-16,0.,-1.));
#16496=DIRECTION('',(0.,-1.,0.));
#16497=DIRECTION('center_axis',(0.,-1.,0.));
#16498=DIRECTION('ref_axis',(-1.85037170770859E-16,0.,-1.));
#16499=DIRECTION('center_axis',(-0.707106781186546,-0.707106781186549,0.));
#16500=DIRECTION('ref_axis',(0.,0.,1.));
#16501=DIRECTION('',(0.,0.,-1.));
#16502=DIRECTION('',(0.707106781186549,-0.707106781186546,0.));
#16503=DIRECTION('',(0.,0.,1.));
#16504=DIRECTION('center_axis',(0.,1.,0.));
#16505=DIRECTION('ref_axis',(-4.16333634234433E-16,0.,-1.));
#16506=DIRECTION('',(3.92523114670945E-16,-0.707106781186548,0.707106781186548));
#16507=DIRECTION('center_axis',(0.,1.,0.));
#16508=DIRECTION('ref_axis',(-4.16333634234433E-16,0.,-1.));
#16509=DIRECTION('center_axis',(0.,-1.,0.));
#16510=DIRECTION('ref_axis',(-4.16333634234433E-16,0.,-1.));
#16511=DIRECTION('center_axis',(0.,-0.707106781186549,-0.707106781186546));
#16512=DIRECTION('ref_axis',(-1.,0.,0.));
#16513=DIRECTION('',(0.,-0.707106781186544,0.707106781186551));
#16514=DIRECTION('',(-1.,0.,0.));
#16515=DIRECTION('',(1.,0.,0.));
#16516=DIRECTION('center_axis',(0.,1.,0.));
#16517=DIRECTION('ref_axis',(1.,0.,0.));
#16518=DIRECTION('',(-0.707106781186548,-0.707106781186548,0.));
#16519=DIRECTION('center_axis',(0.,1.,0.));
#16520=DIRECTION('ref_axis',(1.,0.,0.));
#16521=DIRECTION('center_axis',(0.,-1.,0.));
#16522=DIRECTION('ref_axis',(1.,0.,0.));
#16523=DIRECTION('center_axis',(0.707106781186548,-0.707106781186548,0.));
#16524=DIRECTION('ref_axis',(0.,0.,-1.));
#16525=DIRECTION('',(0.,0.,-1.));
#16526=DIRECTION('',(0.,0.,1.));
#16527=DIRECTION('center_axis',(1.,0.,0.));
#16528=DIRECTION('ref_axis',(0.,0.,1.));
#16529=DIRECTION('',(0.,-1.,0.));
#16530=DIRECTION('',(0.,0.,-1.));
#16531=DIRECTION('',(0.,-1.,0.));
#16532=DIRECTION('',(0.,0.,1.));
#16533=DIRECTION('',(0.,1.,0.));
#16534=DIRECTION('',(0.,0.,-1.));
#16535=DIRECTION('',(0.,-1.,0.));
#16536=DIRECTION('',(0.,0.,1.));
#16537=DIRECTION('',(0.,0.,1.));
#16538=DIRECTION('center_axis',(0.,-1.,0.));
#16539=DIRECTION('ref_axis',(1.,0.,0.));
#16540=DIRECTION('',(0.,-1.,0.));
#16541=DIRECTION('center_axis',(0.,1.,0.));
#16542=DIRECTION('ref_axis',(1.,0.,0.));
#16543=DIRECTION('center_axis',(0.,0.,-1.));
#16544=DIRECTION('ref_axis',(1.,0.,0.));
#16545=DIRECTION('',(0.,-1.,0.));
#16546=DIRECTION('',(-1.,0.,0.));
#16547=DIRECTION('center_axis',(0.,-1.,0.));
#16548=DIRECTION('ref_axis',(-4.16333634234433E-16,0.,-1.));
#16549=DIRECTION('',(0.,-1.,0.));
#16550=DIRECTION('center_axis',(0.,1.,0.));
#16551=DIRECTION('ref_axis',(-4.16333634234433E-16,0.,-1.));
#16552=DIRECTION('center_axis',(-1.,0.,0.));
#16553=DIRECTION('ref_axis',(0.,0.,-1.));
#16554=DIRECTION('',(0.,0.,-1.));
#16555=DIRECTION('',(0.,0.,-1.));
#16556=DIRECTION('',(0.,-1.,0.));
#16557=DIRECTION('',(0.,0.,1.));
#16558=DIRECTION('',(0.,-1.,0.));
#16559=DIRECTION('',(0.,0.,-1.));
#16560=DIRECTION('',(0.,-1.,0.));
#16561=DIRECTION('',(0.,0.,1.));
#16562=DIRECTION('center_axis',(0.707106781186548,-0.707106781186548,0.));
#16563=DIRECTION('ref_axis',(0.,0.,-1.));
#16564=DIRECTION('',(-0.707106781186544,-0.707106781186551,0.));
#16565=DIRECTION('',(0.,0.,-1.));
#16566=DIRECTION('center_axis',(0.,1.,0.));
#16567=DIRECTION('ref_axis',(2.22044604925031E-15,0.,1.));
#16568=DIRECTION('',(0.,-0.707106781186548,-0.707106781186548));
#16569=DIRECTION('center_axis',(0.,1.,0.));
#16570=DIRECTION('ref_axis',(2.22044604925031E-15,0.,1.));
#16571=DIRECTION('center_axis',(0.,-1.,0.));
#16572=DIRECTION('ref_axis',(2.22044604925031E-15,0.,1.));
#16573=DIRECTION('center_axis',(0.,-0.707106781186549,0.707106781186546));
#16574=DIRECTION('ref_axis',(1.,0.,0.));
#16575=DIRECTION('',(0.,-0.707106781186546,-0.707106781186549));
#16576=DIRECTION('',(1.,0.,0.));
#16577=DIRECTION('',(-1.,0.,0.));
#16578=DIRECTION('center_axis',(0.,1.,0.));
#16579=DIRECTION('ref_axis',(-1.,0.,1.11022302462516E-15));
#16580=DIRECTION('',(0.707106781186548,-0.707106781186547,0.));
#16581=DIRECTION('center_axis',(0.,1.,0.));
#16582=DIRECTION('ref_axis',(-1.,0.,1.11022302462516E-15));
#16583=DIRECTION('center_axis',(0.,-1.,0.));
#16584=DIRECTION('ref_axis',(-1.,0.,1.11022302462516E-15));
#16585=DIRECTION('center_axis',(-0.707106781186546,-0.707106781186549,0.));
#16586=DIRECTION('ref_axis',(0.,0.,1.));
#16587=DIRECTION('',(0.,0.,1.));
#16588=DIRECTION('center_axis',(0.,-1.,0.));
#16589=DIRECTION('ref_axis',(-1.,0.,1.11022302462516E-15));
#16590=DIRECTION('',(0.,-1.,0.));
#16591=DIRECTION('center_axis',(0.,1.,0.));
#16592=DIRECTION('ref_axis',(-1.,0.,1.11022302462516E-15));
#16593=DIRECTION('center_axis',(0.,0.,1.));
#16594=DIRECTION('ref_axis',(-1.,0.,0.));
#16595=DIRECTION('',(0.,-1.,0.));
#16596=DIRECTION('',(1.,0.,0.));
#16597=DIRECTION('center_axis',(0.,-1.,0.));
#16598=DIRECTION('ref_axis',(2.22044604925031E-15,0.,1.));
#16599=DIRECTION('center_axis',(0.,1.,0.));
#16600=DIRECTION('ref_axis',(2.22044604925031E-15,0.,1.));
#16601=DIRECTION('center_axis',(0.,-1.,0.));
#16602=DIRECTION('ref_axis',(2.22044604925031E-15,0.,1.));
#16603=DIRECTION('',(-0.707106781186546,0.707106781186549,0.));
#16604=DIRECTION('',(0.,-0.707106781186549,0.707106781186546));
#16605=DIRECTION('center_axis',(0.,1.,0.));
#16606=DIRECTION('ref_axis',(2.22044604925031E-15,0.,1.));
#16607=DIRECTION('center_axis',(0.707106781186549,0.707106781186546,0.));
#16608=DIRECTION('ref_axis',(0.,0.,-1.));
#16609=DIRECTION('',(-0.707106781186546,0.707106781186549,0.));
#16610=DIRECTION('center_axis',(0.,-1.,0.));
#16611=DIRECTION('ref_axis',(1.,0.,0.));
#16612=DIRECTION('',(0.,0.707106781186549,0.707106781186546));
#16613=DIRECTION('center_axis',(0.,0.707106781186548,-0.707106781186547));
#16614=DIRECTION('ref_axis',(-1.,0.,0.));
#16615=DIRECTION('',(0.,0.707106781186547,0.707106781186548));
#16616=DIRECTION('center_axis',(0.,-1.,0.));
#16617=DIRECTION('ref_axis',(-4.16333634234433E-16,0.,-1.));
#16618=DIRECTION('',(0.707106781186547,0.707106781186548,0.));
#16619=DIRECTION('center_axis',(-0.707106781186548,0.707106781186547,0.));
#16620=DIRECTION('ref_axis',(0.,0.,1.));
#16621=DIRECTION('',(0.707106781186547,0.707106781186548,0.));
#16622=DIRECTION('center_axis',(0.,-1.,0.));
#16623=DIRECTION('ref_axis',(-1.,0.,1.11022302462516E-15));
#16624=DIRECTION('',(3.92523114670944E-16,0.707106781186547,-0.707106781186548));
#16625=DIRECTION('center_axis',(0.,1.,0.));
#16626=DIRECTION('ref_axis',(-1.,0.,1.11022302462516E-15));
#16627=DIRECTION('center_axis',(0.,0.707106781186548,0.707106781186547));
#16628=DIRECTION('ref_axis',(1.,0.,0.));
#16629=DIRECTION('',(1.,0.,0.));
#16630=DIRECTION('center_axis',(0.,-1.,0.));
#16631=DIRECTION('ref_axis',(2.22044604925031E-15,0.,1.));
#16632=DIRECTION('',(0.,-1.,0.));
#16633=DIRECTION('center_axis',(0.,-1.,0.));
#16634=DIRECTION('ref_axis',(2.22044604925031E-15,0.,1.));
#16635=DIRECTION('center_axis',(-0.707106781186549,0.,0.707106781186546));
#16636=DIRECTION('ref_axis',(0.707106781186546,0.,0.707106781186549));
#16637=DIRECTION('',(-0.577350269189625,-0.577350269189625,-0.577350269189627));
#16638=DIRECTION('',(0.,1.,0.));
#16639=DIRECTION('',(0.577350269189625,-0.577350269189626,0.577350269189627));
#16640=DIRECTION('center_axis',(0.,0.,-1.));
#16641=DIRECTION('ref_axis',(-1.,0.,0.));
#16642=DIRECTION('',(-1.,0.,0.));
#16643=DIRECTION('',(0.,-1.,0.));
#16644=DIRECTION('',(1.,0.,0.));
#16645=DIRECTION('center_axis',(0.707106781186554,0.,0.707106781186541));
#16646=DIRECTION('ref_axis',(0.707106781186541,0.,-0.707106781186554));
#16647=DIRECTION('',(0.577350269189622,0.577350269189624,-0.577350269189632));
#16648=DIRECTION('',(-0.577350269189622,0.577350269189624,0.577350269189632));
#16649=DIRECTION('center_axis',(0.,1.,0.));
#16650=DIRECTION('ref_axis',(1.,0.,2.46716227694479E-16));
#16651=DIRECTION('',(-0.707106781186548,-0.707106781186548,0.));
#16652=DIRECTION('center_axis',(0.,1.,0.));
#16653=DIRECTION('ref_axis',(1.,0.,2.46716227694479E-16));
#16654=DIRECTION('',(6.28036983473511E-15,0.707106781186546,-0.707106781186549));
#16655=DIRECTION('center_axis',(0.707106781186548,-0.707106781186548,0.));
#16656=DIRECTION('ref_axis',(0.,0.,-1.));
#16657=DIRECTION('',(-0.707106781186551,-0.707106781186544,7.85046229341887E-16));
#16658=DIRECTION('',(0.,0.,-1.));
#16659=DIRECTION('center_axis',(0.,1.,0.));
#16660=DIRECTION('ref_axis',(-4.93432455388959E-16,0.,1.));
#16661=DIRECTION('',(0.,-0.707106781186546,-0.707106781186549));
#16662=DIRECTION('center_axis',(0.,1.,0.));
#16663=DIRECTION('ref_axis',(-4.93432455388959E-16,0.,1.));
#16664=DIRECTION('center_axis',(0.,-0.707106781186549,0.707106781186546));
#16665=DIRECTION('ref_axis',(1.,0.,0.));
#16666=DIRECTION('',(7.85046229341889E-16,-0.707106781186546,-0.707106781186549));
#16667=DIRECTION('',(1.,0.,0.));
#16668=DIRECTION('',(-1.,0.,0.));
#16669=DIRECTION('center_axis',(0.,1.,0.));
#16670=DIRECTION('ref_axis',(-1.,0.,0.));
#16671=DIRECTION('',(0.707106781186548,-0.707106781186547,0.));
#16672=DIRECTION('center_axis',(0.,1.,0.));
#16673=DIRECTION('ref_axis',(-1.,0.,0.));
#16674=DIRECTION('center_axis',(-0.707106781186545,-0.70710678118655,0.));
#16675=DIRECTION('ref_axis',(0.,0.,1.));
#16676=DIRECTION('',(0.70710678118655,-0.707106781186545,-7.85046229341888E-16));
#16677=DIRECTION('',(0.,0.,1.));
#16678=DIRECTION('center_axis',(0.,1.,0.));
#16679=DIRECTION('ref_axis',(-1.85037170770859E-16,0.,-1.));
#16680=DIRECTION('',(0.,-0.707106781186546,0.707106781186549));
#16681=DIRECTION('center_axis',(0.,1.,0.));
#16682=DIRECTION('ref_axis',(-1.85037170770859E-16,0.,-1.));
#16683=DIRECTION('center_axis',(0.,-0.707106781186549,-0.707106781186546));
#16684=DIRECTION('ref_axis',(-1.,0.,0.));
#16685=DIRECTION('',(-1.,0.,0.));
#16686=DIRECTION('',(1.,0.,0.));
#16687=DIRECTION('center_axis',(0.,0.,1.));
#16688=DIRECTION('ref_axis',(-1.,0.,0.));
#16689=DIRECTION('',(1.,0.,0.));
#16690=DIRECTION('center_axis',(0.,1.,0.));
#16691=DIRECTION('ref_axis',(1.,0.,0.));
#16692=DIRECTION('',(0.,0.,-1.));
#16693=DIRECTION('',(-1.,0.,0.));
#16694=DIRECTION('',(0.,0.,1.));
#16695=DIRECTION('',(1.,0.,0.));
#16696=DIRECTION('',(0.,0.,-1.));
#16697=DIRECTION('',(-1.,0.,0.));
#16698=DIRECTION('',(0.,0.,1.));
#16699=DIRECTION('',(1.,0.,0.));
#16700=DIRECTION('',(0.,0.,-1.));
#16701=DIRECTION('',(-1.,0.,0.));
#16702=DIRECTION('',(0.,0.,1.));
#16703=DIRECTION('',(1.,0.,0.));
#16704=DIRECTION('',(0.,0.,-1.));
#16705=DIRECTION('',(-1.,0.,0.));
#16706=DIRECTION('',(0.,0.,1.));
#16707=DIRECTION('',(1.,0.,0.));
#16708=DIRECTION('center_axis',(-0.707106781186548,-0.707106781186547,0.));
#16709=DIRECTION('ref_axis',(0.,0.,1.));
#16710=DIRECTION('',(0.,0.,1.));
#16711=DIRECTION('',(-0.707106781186547,0.707106781186548,0.));
#16712=DIRECTION('center_axis',(0.,1.,0.));
#16713=DIRECTION('ref_axis',(-1.,0.,1.11022302462516E-15));
#16714=DIRECTION('',(-3.92523114670943E-16,0.707106781186547,0.707106781186547));
#16715=DIRECTION('center_axis',(0.,-1.,0.));
#16716=DIRECTION('ref_axis',(-1.,0.,1.11022302462516E-15));
#16717=DIRECTION('center_axis',(0.,1.,0.));
#16718=DIRECTION('ref_axis',(-1.,0.,1.11022302462516E-15));
#16719=DIRECTION('center_axis',(0.,-0.707106781186548,0.707106781186548));
#16720=DIRECTION('ref_axis',(1.,0.,0.));
#16721=DIRECTION('',(0.,0.707106781186547,0.707106781186547));
#16722=DIRECTION('',(-1.,0.,0.));
#16723=DIRECTION('',(1.,0.,0.));
#16724=DIRECTION('center_axis',(0.,1.,0.));
#16725=DIRECTION('ref_axis',(2.22044604925031E-15,0.,1.));
#16726=DIRECTION('',(0.707106781186546,0.707106781186549,0.));
#16727=DIRECTION('center_axis',(0.,1.,0.));
#16728=DIRECTION('ref_axis',(2.22044604925031E-15,0.,1.));
#16729=DIRECTION('center_axis',(0.707106781186549,-0.707106781186546,0.));
#16730=DIRECTION('ref_axis',(0.,0.,-1.));
#16731=DIRECTION('',(0.,0.,-1.));
#16732=DIRECTION('center_axis',(0.,1.,0.));
#16733=DIRECTION('ref_axis',(1.,0.,0.));
#16734=DIRECTION('center_axis',(0.707106781186549,0.707106781186546,0.));
#16735=DIRECTION('ref_axis',(0.,0.,-1.));
#16736=DIRECTION('',(0.,0.,1.));
#16737=DIRECTION('',(0.707106781186543,-0.707106781186552,0.));
#16738=DIRECTION('center_axis',(0.,-1.,0.));
#16739=DIRECTION('ref_axis',(2.22044604925031E-15,0.,1.));
#16740=DIRECTION('',(0.,-0.707106781186549,0.707106781186546));
#16741=DIRECTION('center_axis',(0.,-1.,0.));
#16742=DIRECTION('ref_axis',(2.22044604925031E-15,0.,1.));
#16743=DIRECTION('center_axis',(0.,0.707106781186548,0.707106781186548));
#16744=DIRECTION('ref_axis',(1.,0.,0.));
#16745=DIRECTION('',(0.,-0.707106781186547,0.707106781186547));
#16746=DIRECTION('',(-1.,0.,0.));
#16747=DIRECTION('center_axis',(0.,-1.,0.));
#16748=DIRECTION('ref_axis',(-1.,0.,1.11022302462516E-15));
#16749=DIRECTION('',(-0.707106781186546,-0.707106781186549,0.));
#16750=DIRECTION('center_axis',(0.,-1.,0.));
#16751=DIRECTION('ref_axis',(-1.,0.,1.11022302462516E-15));
#16752=DIRECTION('center_axis',(-0.707106781186547,0.707106781186548,0.));
#16753=DIRECTION('ref_axis',(0.,0.,1.));
#16754=DIRECTION('',(0.,0.,-1.));
#16755=DIRECTION('center_axis',(0.,-1.,0.));
#16756=DIRECTION('ref_axis',(-1.,0.,0.));
#16757=DIRECTION('center_axis',(-0.707106781186554,-0.707106781186541,0.));
#16758=DIRECTION('ref_axis',(0.,0.,1.));
#16759=DIRECTION('',(-0.577350269189622,0.577350269189632,-0.577350269189624));
#16760=DIRECTION('',(0.,0.,-1.));
#16761=DIRECTION('',(-0.577350269189622,0.577350269189632,0.577350269189623));
#16762=DIRECTION('center_axis',(0.707106781186554,-0.707106781186541,0.));
#16763=DIRECTION('ref_axis',(0.,0.,-1.));
#16764=DIRECTION('',(0.577350269189622,0.577350269189632,0.577350269189624));
#16765=DIRECTION('',(0.,0.,1.));
#16766=DIRECTION('',(-0.577350269189622,-0.577350269189632,0.577350269189624));
#16767=DIRECTION('center_axis',(0.,-0.707106781186543,0.707106781186552));
#16768=DIRECTION('ref_axis',(1.,0.,0.));
#16769=DIRECTION('',(-1.,0.,0.));
#16770=DIRECTION('center_axis',(0.,-0.707106781186543,-0.707106781186552));
#16771=DIRECTION('ref_axis',(-1.,0.,0.));
#16772=DIRECTION('',(1.,0.,0.));
#16773=DIRECTION('center_axis',(0.,0.,1.));
#16774=DIRECTION('ref_axis',(1.,0.,0.));
#16775=DIRECTION('',(0.,1.,0.));
#16776=DIRECTION('',(1.,0.,0.));
#16777=DIRECTION('',(0.,1.,0.));
#16778=DIRECTION('center_axis',(-1.,0.,0.));
#16779=DIRECTION('ref_axis',(0.,0.,1.));
#16780=DIRECTION('',(0.,1.,0.));
#16781=DIRECTION('',(0.,0.,1.));
#16782=DIRECTION('center_axis',(-1.,0.,0.));
#16783=DIRECTION('ref_axis',(0.,0.,-1.));
#16784=DIRECTION('center_axis',(-0.707106781186553,-0.707106781186542,0.));
#16785=DIRECTION('ref_axis',(0.,0.,1.));
#16786=DIRECTION('',(-0.577350269189623,0.577350269189631,-0.577350269189623));
#16787=DIRECTION('',(0.,0.,-1.));
#16788=DIRECTION('',(-0.577350269189623,0.577350269189632,0.577350269189623));
#16789=DIRECTION('center_axis',(0.707106781186553,-0.707106781186542,0.));
#16790=DIRECTION('ref_axis',(0.,0.,-1.));
#16791=DIRECTION('',(0.577350269189622,0.577350269189631,0.577350269189624));
#16792=DIRECTION('',(0.,0.,1.));
#16793=DIRECTION('',(-0.577350269189622,-0.577350269189631,0.577350269189624));
#16794=DIRECTION('center_axis',(0.,-0.707106781186543,0.707106781186552));
#16795=DIRECTION('ref_axis',(1.,0.,0.));
#16796=DIRECTION('',(-1.,0.,0.));
#16797=DIRECTION('center_axis',(0.,-0.707106781186543,-0.707106781186552));
#16798=DIRECTION('ref_axis',(-1.,0.,0.));
#16799=DIRECTION('',(1.,0.,0.));
#16800=DIRECTION('center_axis',(0.,0.,1.));
#16801=DIRECTION('ref_axis',(1.,0.,0.));
#16802=DIRECTION('',(0.,1.,0.));
#16803=DIRECTION('',(1.,0.,0.));
#16804=DIRECTION('',(0.,1.,0.));
#16805=DIRECTION('center_axis',(-1.,0.,0.));
#16806=DIRECTION('ref_axis',(0.,0.,1.));
#16807=DIRECTION('',(0.,1.,0.));
#16808=DIRECTION('',(0.,0.,1.));
#16809=DIRECTION('center_axis',(-1.,0.,0.));
#16810=DIRECTION('ref_axis',(0.,0.,-1.));
#16811=DIRECTION('center_axis',(-0.707106781186551,-0.707106781186544,0.));
#16812=DIRECTION('ref_axis',(0.,0.,1.));
#16813=DIRECTION('',(-0.577350269189625,0.57735026918963,-0.577350269189622));
#16814=DIRECTION('',(0.,0.,-1.));
#16815=DIRECTION('',(-0.577350269189625,0.577350269189631,0.577350269189622));
#16816=DIRECTION('center_axis',(0.707106781186552,-0.707106781186543,0.));
#16817=DIRECTION('ref_axis',(0.,0.,-1.));
#16818=DIRECTION('',(0.577350269189623,0.577350269189631,0.577350269189623));
#16819=DIRECTION('',(0.,0.,1.));
#16820=DIRECTION('',(-0.577350269189623,-0.577350269189631,0.577350269189623));
#16821=DIRECTION('center_axis',(0.,-0.707106781186543,0.707106781186552));
#16822=DIRECTION('ref_axis',(1.,0.,0.));
#16823=DIRECTION('',(-1.,0.,0.));
#16824=DIRECTION('center_axis',(0.,-0.707106781186543,-0.707106781186552));
#16825=DIRECTION('ref_axis',(-1.,0.,0.));
#16826=DIRECTION('',(1.,0.,0.));
#16827=DIRECTION('center_axis',(0.,0.,1.));
#16828=DIRECTION('ref_axis',(1.,0.,0.));
#16829=DIRECTION('',(0.,1.,0.));
#16830=DIRECTION('',(1.,0.,0.));
#16831=DIRECTION('',(0.,1.,0.));
#16832=DIRECTION('center_axis',(-1.,0.,0.));
#16833=DIRECTION('ref_axis',(0.,0.,1.));
#16834=DIRECTION('',(0.,1.,0.));
#16835=DIRECTION('',(0.,0.,1.));
#16836=DIRECTION('center_axis',(-1.,0.,0.));
#16837=DIRECTION('ref_axis',(0.,0.,-1.));
#16838=DIRECTION('center_axis',(-0.707106781186554,-0.707106781186541,0.));
#16839=DIRECTION('ref_axis',(0.,0.,1.));
#16840=DIRECTION('',(-0.577350269189622,0.577350269189632,-0.577350269189624));
#16841=DIRECTION('',(0.,0.,-1.));
#16842=DIRECTION('',(-0.577350269189622,0.577350269189632,0.577350269189623));
#16843=DIRECTION('center_axis',(0.707106781186552,-0.707106781186543,0.));
#16844=DIRECTION('ref_axis',(0.,0.,-1.));
#16845=DIRECTION('',(0.577350269189623,0.577350269189631,0.577350269189623));
#16846=DIRECTION('',(0.,0.,1.));
#16847=DIRECTION('',(-0.577350269189623,-0.577350269189631,0.577350269189623));
#16848=DIRECTION('center_axis',(0.,-0.707106781186543,0.707106781186552));
#16849=DIRECTION('ref_axis',(1.,0.,0.));
#16850=DIRECTION('',(-1.,0.,0.));
#16851=DIRECTION('center_axis',(0.,-0.707106781186543,-0.707106781186552));
#16852=DIRECTION('ref_axis',(-1.,0.,0.));
#16853=DIRECTION('',(1.,0.,0.));
#16854=DIRECTION('center_axis',(0.,0.,1.));
#16855=DIRECTION('ref_axis',(1.,0.,0.));
#16856=DIRECTION('',(0.,1.,0.));
#16857=DIRECTION('',(1.,0.,0.));
#16858=DIRECTION('',(0.,1.,0.));
#16859=DIRECTION('center_axis',(-1.,0.,0.));
#16860=DIRECTION('ref_axis',(0.,0.,1.));
#16861=DIRECTION('',(0.,1.,0.));
#16862=DIRECTION('',(0.,0.,1.));
#16863=DIRECTION('center_axis',(-1.,0.,0.));
#16864=DIRECTION('ref_axis',(0.,0.,-1.));
#16865=DIRECTION('center_axis',(-1.,0.,0.));
#16866=DIRECTION('ref_axis',(0.,0.,-1.));
#16867=DIRECTION('',(-1.,0.,0.));
#16868=DIRECTION('center_axis',(1.,0.,0.));
#16869=DIRECTION('ref_axis',(0.,0.,-1.));
#16870=DIRECTION('center_axis',(-1.,0.,0.));
#16871=DIRECTION('ref_axis',(0.,0.,-1.));
#16872=DIRECTION('',(-1.,0.,0.));
#16873=DIRECTION('center_axis',(1.,0.,0.));
#16874=DIRECTION('ref_axis',(0.,0.,-1.));
#16875=DIRECTION('center_axis',(-1.,0.,0.));
#16876=DIRECTION('ref_axis',(0.,0.,-1.));
#16877=DIRECTION('',(-1.,0.,0.));
#16878=DIRECTION('center_axis',(1.,0.,0.));
#16879=DIRECTION('ref_axis',(0.,0.,-1.));
#16880=DIRECTION('center_axis',(-1.,0.,0.));
#16881=DIRECTION('ref_axis',(0.,0.,-1.));
#16882=DIRECTION('',(-1.,0.,0.));
#16883=DIRECTION('center_axis',(1.,0.,0.));
#16884=DIRECTION('ref_axis',(0.,0.,-1.));
#16885=DIRECTION('center_axis',(-1.,0.,0.));
#16886=DIRECTION('ref_axis',(0.,0.,-1.));
#16887=DIRECTION('',(-1.,0.,0.));
#16888=DIRECTION('center_axis',(0.,0.,-1.));
#16889=DIRECTION('ref_axis',(-1.,0.,0.));
#16890=DIRECTION('',(0.,1.,0.));
#16891=DIRECTION('',(-1.,0.,0.));
#16892=DIRECTION('center_axis',(1.,0.,0.));
#16893=DIRECTION('ref_axis',(0.,0.,-1.));
#16894=DIRECTION('',(0.,0.,-1.));
#16895=DIRECTION('center_axis',(0.,1.,0.));
#16896=DIRECTION('ref_axis',(0.,0.,1.));
#16897=DIRECTION('center_axis',(0.,0.,-1.));
#16898=DIRECTION('ref_axis',(-1.,0.,0.));
#16899=DIRECTION('',(0.,1.,0.));
#16900=DIRECTION('',(-1.,0.,0.));
#16901=DIRECTION('center_axis',(1.,0.,0.));
#16902=DIRECTION('ref_axis',(0.,0.,-1.));
#16903=DIRECTION('',(0.,0.,-1.));
#16904=DIRECTION('center_axis',(0.,1.,0.));
#16905=DIRECTION('ref_axis',(0.,0.,1.));
#16906=DIRECTION('center_axis',(0.,0.,-1.));
#16907=DIRECTION('ref_axis',(-1.,0.,0.));
#16908=DIRECTION('',(0.,1.,0.));
#16909=DIRECTION('',(-1.,0.,0.));
#16910=DIRECTION('center_axis',(1.,0.,0.));
#16911=DIRECTION('ref_axis',(0.,0.,-1.));
#16912=DIRECTION('',(0.,0.,-1.));
#16913=DIRECTION('center_axis',(0.,1.,0.));
#16914=DIRECTION('ref_axis',(0.,0.,1.));
#16915=DIRECTION('center_axis',(0.,0.,-1.));
#16916=DIRECTION('ref_axis',(-1.,0.,0.));
#16917=DIRECTION('',(0.,1.,0.));
#16918=DIRECTION('',(-1.,0.,0.));
#16919=DIRECTION('center_axis',(1.,0.,0.));
#16920=DIRECTION('ref_axis',(0.,0.,-1.));
#16921=DIRECTION('',(0.,0.,-1.));
#16922=DIRECTION('center_axis',(0.,1.,0.));
#16923=DIRECTION('ref_axis',(0.,0.,1.));
#16924=DIRECTION('center_axis',(0.,0.,1.));
#16925=DIRECTION('ref_axis',(-1.,0.,0.));
#16926=DIRECTION('',(0.,-1.,0.));
#16927=DIRECTION('center_axis',(0.,-1.,0.));
#16928=DIRECTION('ref_axis',(-1.,0.,1.11022302462516E-15));
#16929=DIRECTION('center_axis',(0.,1.,0.));
#16930=DIRECTION('ref_axis',(1.,0.,0.));
#16931=DIRECTION('center_axis',(0.,1.,0.));
#16932=DIRECTION('ref_axis',(1.,0.,0.));
#16933=DIRECTION('center_axis',(0.,1.,0.));
#16934=DIRECTION('ref_axis',(1.,0.,0.));
#16935=DIRECTION('center_axis',(0.,0.,-1.));
#16936=DIRECTION('ref_axis',(1.,0.,0.));
#16937=DIRECTION('',(-1.,0.,0.));
#16938=DIRECTION('center_axis',(0.,1.,0.));
#16939=DIRECTION('ref_axis',(1.,0.,0.));
#16940=DIRECTION('center_axis',(0.,1.,0.));
#16941=DIRECTION('ref_axis',(1.,0.,0.));
#25937=CARTESIAN_POINT('',(0.,0.,0.));
#25938=CARTESIAN_POINT('Origin',(28.2,-32.15,4.));
#25939=CARTESIAN_POINT('',(34.,-31.9,10.2136945531624));
#25940=CARTESIAN_POINT('',(34.,-32.4,10.8818602136341));
#25941=CARTESIAN_POINT('Ctrl Pts',(34.,-32.4,10.8818602136341));
#25942=CARTESIAN_POINT('Ctrl Pts',(34.,-32.1372444185762,10.5382321596773));
#25943=CARTESIAN_POINT('Ctrl Pts',(34.,-31.9,10.2136945531624));
#25944=CARTESIAN_POINT('',(37.2,-32.4,4.));
#25945=CARTESIAN_POINT('Origin',(28.2,-32.4,4.));
#25946=CARTESIAN_POINT('',(36.7,-31.9,4.));
#25947=CARTESIAN_POINT('',(37.2,-32.4,4.));
#25948=CARTESIAN_POINT('Origin',(28.2,-31.9,4.));
#25949=CARTESIAN_POINT('Origin',(36.95,-32.15,-2.));
#25950=CARTESIAN_POINT('',(37.2,-32.4,-4.));
#25951=CARTESIAN_POINT('',(37.2,-32.4,-2.));
#25952=CARTESIAN_POINT('',(36.7,-31.9,-4.));
#25953=CARTESIAN_POINT('',(37.2,-32.4,-4.));
#25954=CARTESIAN_POINT('',(36.7,-31.9,-2.));
#25955=CARTESIAN_POINT('Origin',(28.2,-32.15,-4.));
#25956=CARTESIAN_POINT('',(34.,-32.4,-10.8818602136341));
#25957=CARTESIAN_POINT('',(34.,-31.9,-10.2136945531624));
#25958=CARTESIAN_POINT('Ctrl Pts',(34.,-31.9,-10.2136945531624));
#25959=CARTESIAN_POINT('Ctrl Pts',(34.,-32.1372444185762,-10.5382321596772));
#25960=CARTESIAN_POINT('Ctrl Pts',(34.,-32.4,-10.8818602136341));
#25961=CARTESIAN_POINT('Origin',(28.2,-31.9,-4.));
#25962=CARTESIAN_POINT('Origin',(28.2,-32.4,-4.));
#25963=CARTESIAN_POINT('Origin',(28.2,-31.9,-4.));
#25964=CARTESIAN_POINT('',(34.,-31.4,-10.8818602136341));
#25965=CARTESIAN_POINT('',(34.,-31.9,-10.8818602136341));
#25966=CARTESIAN_POINT('',(37.2,-69.5,-4.));
#25967=CARTESIAN_POINT('',(37.2,-31.9,-4.));
#25968=CARTESIAN_POINT('',(28.2,-69.5,-13.));
#25969=CARTESIAN_POINT('Origin',(28.2,-69.5,-4.));
#25970=CARTESIAN_POINT('',(28.2,-31.9,-13.));
#25971=CARTESIAN_POINT('',(28.2,-31.9,-13.));
#25972=CARTESIAN_POINT('',(33.5,-31.9,-11.2739260375673));
#25973=CARTESIAN_POINT('Origin',(28.2,-31.9,-4.));
#25974=CARTESIAN_POINT('Origin',(28.2,-37.2,-4.));
#25975=CARTESIAN_POINT('Origin',(37.2,-31.9,-4.));
#25976=CARTESIAN_POINT('',(37.2,-69.5,4.));
#25977=CARTESIAN_POINT('',(37.2,-31.9,4.));
#25978=CARTESIAN_POINT('',(37.2,-69.5,-2.));
#25979=CARTESIAN_POINT('',(37.2,-61.,1.525));
#25980=CARTESIAN_POINT('Origin',(37.2,-61.,0.));
#25981=CARTESIAN_POINT('Origin',(28.2,-31.9,4.));
#25982=CARTESIAN_POINT('',(34.,-31.4,10.8818602136341));
#25983=CARTESIAN_POINT('',(34.,-31.9,10.8818602136341));
#25984=CARTESIAN_POINT('',(33.5,-31.9,11.2739260375673));
#25985=CARTESIAN_POINT('Origin',(28.2,-37.2,4.));
#25986=CARTESIAN_POINT('',(28.2,-31.9,13.));
#25987=CARTESIAN_POINT('Origin',(28.2,-31.9,4.));
#25988=CARTESIAN_POINT('',(28.2,-69.5,13.));
#25989=CARTESIAN_POINT('',(28.2,-31.9,13.));
#25990=CARTESIAN_POINT('Origin',(28.2,-69.5,4.));
#25991=CARTESIAN_POINT('Origin',(15.2,-0.25,0.));
#25992=CARTESIAN_POINT('',(9.85,0.,6.55186037543834E-16));
#25993=CARTESIAN_POINT('Origin',(15.2,0.,0.));
#25994=CARTESIAN_POINT('',(10.35,-0.5,-5.93953697586466E-16));
#25995=CARTESIAN_POINT('',(10.1,-0.25,6.2456986756515E-16));
#25996=CARTESIAN_POINT('Origin',(15.2,-0.5,0.));
#25997=CARTESIAN_POINT('Origin',(15.2,0.,-2.22044604925031E-15));
#25998=CARTESIAN_POINT('',(33.5,0.,16.8));
#25999=CARTESIAN_POINT('',(32.,0.,18.3));
#26000=CARTESIAN_POINT('Origin',(32.,0.,16.8));
#26001=CARTESIAN_POINT('',(33.5,0.,-16.8));
#26002=CARTESIAN_POINT('',(33.5,0.,-8.4));
#26003=CARTESIAN_POINT('',(32.,0.,-18.3));
#26004=CARTESIAN_POINT('Origin',(32.,0.,-16.8));
#26005=CARTESIAN_POINT('',(-1.6,0.,-18.3));
#26006=CARTESIAN_POINT('',(6.8,0.,-18.3));
#26007=CARTESIAN_POINT('',(-3.1,0.,-16.8));
#26008=CARTESIAN_POINT('Origin',(-1.6,0.,-16.8));
#26009=CARTESIAN_POINT('',(-3.1,0.,16.8));
#26010=CARTESIAN_POINT('',(-3.1,0.,8.4));
#26011=CARTESIAN_POINT('',(-1.6,0.,18.3));
#26012=CARTESIAN_POINT('Origin',(-1.6,0.,16.8));
#26013=CARTESIAN_POINT('',(23.6,0.,18.3));
#26014=CARTESIAN_POINT('Origin',(15.2,0.,0.));
#26015=CARTESIAN_POINT('',(10.35,-32.5,5.93953697586466E-16));
#26016=CARTESIAN_POINT('',(10.35,0.,-5.93953697586466E-16));
#26017=CARTESIAN_POINT('Origin',(15.2,-32.5,0.));
#26018=CARTESIAN_POINT('Origin',(2.2,-32.15,-4.));
#26019=CARTESIAN_POINT('',(-3.6,-31.9,-10.2136945531624));
#26020=CARTESIAN_POINT('',(-3.6,-32.4,-10.8818602136341));
#26021=CARTESIAN_POINT('Ctrl Pts',(-3.6,-32.4,-10.8818602136341));
#26022=CARTESIAN_POINT('Ctrl Pts',(-3.6,-32.1372444185762,-10.5382321596773));
#26023=CARTESIAN_POINT('Ctrl Pts',(-3.6,-31.9,-10.2136945531624));
#26024=CARTESIAN_POINT('',(-6.8,-32.4,-4.));
#26025=CARTESIAN_POINT('Origin',(2.2,-32.4,-4.));
#26026=CARTESIAN_POINT('',(-6.3,-31.9,-4.));
#26027=CARTESIAN_POINT('',(-6.8,-32.4,-4.));
#26028=CARTESIAN_POINT('Origin',(2.2,-31.9,-4.));
#26029=CARTESIAN_POINT('Origin',(-6.55,-32.15,2.));
#26030=CARTESIAN_POINT('',(-6.8,-32.4,4.));
#26031=CARTESIAN_POINT('',(-6.8,-32.4,2.));
#26032=CARTESIAN_POINT('',(-6.3,-31.9,4.));
#26033=CARTESIAN_POINT('',(-6.8,-32.4,4.));
#26034=CARTESIAN_POINT('',(-6.3,-31.9,2.));
#26035=CARTESIAN_POINT('Origin',(2.2,-32.15,4.));
#26036=CARTESIAN_POINT('',(-3.6,-32.4,10.8818602136341));
#26037=CARTESIAN_POINT('',(-3.6,-31.9,10.2136945531624));
#26038=CARTESIAN_POINT('Ctrl Pts',(-3.6,-31.9,10.2136945531624));
#26039=CARTESIAN_POINT('Ctrl Pts',(-3.6,-32.1372444185762,10.5382321596772));
#26040=CARTESIAN_POINT('Ctrl Pts',(-3.6,-32.4,10.8818602136341));
#26041=CARTESIAN_POINT('Origin',(2.2,-31.9,4.));
#26042=CARTESIAN_POINT('Origin',(2.2,-32.4,4.));
#26043=CARTESIAN_POINT('Origin',(2.2,-31.9,4.));
#26044=CARTESIAN_POINT('',(-3.6,-31.4,10.8818602136341));
#26045=CARTESIAN_POINT('',(-3.6,-31.9,10.8818602136341));
#26046=CARTESIAN_POINT('',(-6.8,-69.5,4.));
#26047=CARTESIAN_POINT('',(-6.8,-31.9,4.));
#26048=CARTESIAN_POINT('',(2.2,-69.5,13.));
#26049=CARTESIAN_POINT('Origin',(2.2,-69.5,4.));
#26050=CARTESIAN_POINT('',(2.2,-31.9,13.));
#26051=CARTESIAN_POINT('',(2.2,-31.9,13.));
#26052=CARTESIAN_POINT('',(-3.1,-31.9,11.2739260375673));
#26053=CARTESIAN_POINT('Origin',(2.2,-31.9,4.));
#26054=CARTESIAN_POINT('Origin',(2.2,-37.2,4.));
#26055=CARTESIAN_POINT('Origin',(-6.8,-31.9,4.));
#26056=CARTESIAN_POINT('',(-6.8,-69.5,-4.));
#26057=CARTESIAN_POINT('',(-6.8,-31.9,-4.));
#26058=CARTESIAN_POINT('',(-6.8,-69.5,2.));
#26059=CARTESIAN_POINT('',(-6.8,-61.,1.525));
#26060=CARTESIAN_POINT('Origin',(-6.8,-61.,0.));
#26061=CARTESIAN_POINT('Origin',(2.2,-31.9,-4.));
#26062=CARTESIAN_POINT('',(-3.6,-31.4,-10.8818602136341));
#26063=CARTESIAN_POINT('',(-3.6,-31.9,-10.8818602136341));
#26064=CARTESIAN_POINT('',(-3.1,-31.9,-11.2739260375673));
#26065=CARTESIAN_POINT('Origin',(2.2,-37.2,-4.));
#26066=CARTESIAN_POINT('',(2.2,-31.9,-13.));
#26067=CARTESIAN_POINT('Origin',(2.2,-31.9,-4.));
#26068=CARTESIAN_POINT('',(2.2,-69.5,-13.));
#26069=CARTESIAN_POINT('',(2.2,-31.9,-13.));
#26070=CARTESIAN_POINT('Origin',(2.2,-69.5,-4.));
#26071=CARTESIAN_POINT('Origin',(-3.35,-31.65,8.4));
#26072=CARTESIAN_POINT('',(-3.6,-31.4,-16.8));
#26073=CARTESIAN_POINT('',(-3.6,-31.4,8.4));
#26074=CARTESIAN_POINT('',(-3.1,-31.9,-16.8));
#26075=CARTESIAN_POINT('',(-3.6,-31.4,-16.8));
#26076=CARTESIAN_POINT('',(-3.1,-31.9,8.4));
#26077=CARTESIAN_POINT('Origin',(-1.6,-31.65,-16.8));
#26078=CARTESIAN_POINT('',(-1.6,-31.4,-18.8));
#26079=CARTESIAN_POINT('',(-1.6,-31.9,-18.3));
#26080=CARTESIAN_POINT('',(-1.6,-31.4,-18.8));
#26081=CARTESIAN_POINT('Origin',(-1.6,-31.9,-16.8));
#26082=CARTESIAN_POINT('Origin',(-1.6,-31.4,-16.8));
#26083=CARTESIAN_POINT('Origin',(6.8,-31.65,-18.55));
#26084=CARTESIAN_POINT('',(32.,-31.4,-18.8));
#26085=CARTESIAN_POINT('',(32.,-31.9,-18.3));
#26086=CARTESIAN_POINT('',(32.,-31.4,-18.8));
#26087=CARTESIAN_POINT('',(6.8,-31.9,-18.3));
#26088=CARTESIAN_POINT('',(6.8,-31.4,-18.8));
#26089=CARTESIAN_POINT('Origin',(32.,-31.65,-16.8));
#26090=CARTESIAN_POINT('',(34.,-31.4,-16.8));
#26091=CARTESIAN_POINT('',(33.5,-31.9,-16.8));
#26092=CARTESIAN_POINT('',(34.,-31.4,-16.8));
#26093=CARTESIAN_POINT('Origin',(32.,-31.9,-16.8));
#26094=CARTESIAN_POINT('Origin',(32.,-31.4,-16.8));
#26095=CARTESIAN_POINT('Origin',(33.75,-31.65,-8.4));
#26096=CARTESIAN_POINT('',(33.5,-31.9,-8.4));
#26097=CARTESIAN_POINT('',(34.,-31.4,-8.4));
#26098=CARTESIAN_POINT('Origin',(34.,0.,-16.8));
#26099=CARTESIAN_POINT('',(34.,-0.5,-16.8));
#26100=CARTESIAN_POINT('',(34.,0.,-16.8));
#26101=CARTESIAN_POINT('',(34.,-0.5,16.8));
#26102=CARTESIAN_POINT('',(34.,-0.5,-8.4));
#26103=CARTESIAN_POINT('',(34.,-12.5,16.8));
#26104=CARTESIAN_POINT('',(34.,0.,16.8));
#26105=CARTESIAN_POINT('',(34.,-12.5,15.3));
#26106=CARTESIAN_POINT('',(34.,-12.5,1.));
#26107=CARTESIAN_POINT('',(34.,-19.5,15.3));
#26108=CARTESIAN_POINT('',(34.,-8.,15.3));
#26109=CARTESIAN_POINT('',(34.,-19.5,16.8));
#26110=CARTESIAN_POINT('',(34.,-19.5,1.));
#26111=CARTESIAN_POINT('',(34.,-31.4,16.8));
#26112=CARTESIAN_POINT('',(34.,0.,16.8));
#26113=CARTESIAN_POINT('',(34.,-31.4,-8.4));
#26114=CARTESIAN_POINT('',(34.,-31.9,-16.8));
#26115=CARTESIAN_POINT('Origin',(32.,0.,-16.8));
#26116=CARTESIAN_POINT('',(32.,-0.5,-18.8));
#26117=CARTESIAN_POINT('',(32.,0.,-18.8));
#26118=CARTESIAN_POINT('Origin',(32.,-0.5,-16.8));
#26119=CARTESIAN_POINT('Origin',(-1.6,0.,-18.8));
#26120=CARTESIAN_POINT('',(-1.6,-0.5,-18.8));
#26121=CARTESIAN_POINT('',(-1.6,0.,-18.8));
#26122=CARTESIAN_POINT('',(6.8,-0.5,-18.8));
#26123=CARTESIAN_POINT('Origin',(-1.6,0.,-16.8));
#26124=CARTESIAN_POINT('',(-3.6,-0.5,-16.8));
#26125=CARTESIAN_POINT('',(-3.6,0.,-16.8));
#26126=CARTESIAN_POINT('Origin',(-1.6,-0.5,-16.8));
#26127=CARTESIAN_POINT('Origin',(-3.6,0.,16.8));
#26128=CARTESIAN_POINT('',(-3.6,-31.9,16.8));
#26129=CARTESIAN_POINT('',(-3.6,-31.4,16.8));
#26130=CARTESIAN_POINT('',(-3.6,-31.4,8.4));
#26131=CARTESIAN_POINT('',(-3.6,-19.5,16.8));
#26132=CARTESIAN_POINT('',(-3.6,0.,16.8));
#26133=CARTESIAN_POINT('',(-3.6,-19.5,15.3));
#26134=CARTESIAN_POINT('',(-3.6,-19.5,17.8));
#26135=CARTESIAN_POINT('',(-3.6,-12.5,15.3));
#26136=CARTESIAN_POINT('',(-3.6,-8.,15.3));
#26137=CARTESIAN_POINT('',(-3.6,-12.5,16.8));
#26138=CARTESIAN_POINT('',(-3.6,-12.5,17.8));
#26139=CARTESIAN_POINT('',(-3.6,-0.5,16.8));
#26140=CARTESIAN_POINT('',(-3.6,0.,16.8));
#26141=CARTESIAN_POINT('',(-3.6,-0.5,8.4));
#26142=CARTESIAN_POINT('Origin',(33.75,-31.65,-8.4));
#26143=CARTESIAN_POINT('',(33.5,-31.9,16.8));
#26144=CARTESIAN_POINT('',(34.,-31.4,16.8));
#26145=CARTESIAN_POINT('',(33.5,-31.9,-8.4));
#26146=CARTESIAN_POINT('Origin',(32.,-31.65,16.8));
#26147=CARTESIAN_POINT('',(32.,-31.4,18.8));
#26148=CARTESIAN_POINT('',(32.,-31.9,18.3));
#26149=CARTESIAN_POINT('',(32.,-31.4,18.8));
#26150=CARTESIAN_POINT('Origin',(32.,-31.9,16.8));
#26151=CARTESIAN_POINT('Origin',(32.,-31.4,16.8));
#26152=CARTESIAN_POINT('Origin',(23.6,-31.65,18.55));
#26153=CARTESIAN_POINT('',(-1.6,-31.4,18.8));
#26154=CARTESIAN_POINT('',(-1.6,-31.9,18.3));
#26155=CARTESIAN_POINT('',(-1.6,-31.4,18.8));
#26156=CARTESIAN_POINT('',(23.6,-31.9,18.3));
#26157=CARTESIAN_POINT('',(23.6,-31.4,18.8));
#26158=CARTESIAN_POINT('Origin',(-1.6,-31.65,16.8));
#26159=CARTESIAN_POINT('',(-3.1,-31.9,16.8));
#26160=CARTESIAN_POINT('',(-3.6,-31.4,16.8));
#26161=CARTESIAN_POINT('Origin',(-1.6,-31.9,16.8));
#26162=CARTESIAN_POINT('Origin',(-1.6,-31.4,16.8));
#26163=CARTESIAN_POINT('Origin',(-3.35,-31.65,8.4));
#26164=CARTESIAN_POINT('',(-3.1,-31.9,8.4));
#26165=CARTESIAN_POINT('Origin',(-1.6,0.,16.8));
#26166=CARTESIAN_POINT('',(-1.6,-19.5,18.8));
#26167=CARTESIAN_POINT('',(-1.6,0.,18.8));
#26168=CARTESIAN_POINT('Origin',(-1.6,-19.5,16.8));
#26169=CARTESIAN_POINT('Origin',(32.,0.,18.8));
#26170=CARTESIAN_POINT('',(32.,-19.5,18.8));
#26171=CARTESIAN_POINT('',(32.,0.,18.8));
#26172=CARTESIAN_POINT('',(33.6,-19.5,18.8));
#26173=CARTESIAN_POINT('Origin',(32.,0.,16.8));
#26174=CARTESIAN_POINT('Origin',(32.,-19.5,16.8));
#26175=CARTESIAN_POINT('Origin',(32.,-0.25,16.8));
#26176=CARTESIAN_POINT('',(34.,-0.5,16.8));
#26177=CARTESIAN_POINT('',(32.,-0.5,18.8));
#26178=CARTESIAN_POINT('',(32.,0.,18.3));
#26179=CARTESIAN_POINT('Origin',(32.,-0.5,16.8));
#26180=CARTESIAN_POINT('Origin',(33.75,-0.25,-8.4));
#26181=CARTESIAN_POINT('',(34.,-0.5,-16.8));
#26182=CARTESIAN_POINT('Origin',(32.,-0.25,-16.8));
#26183=CARTESIAN_POINT('',(32.,-0.5,-18.8));
#26184=CARTESIAN_POINT('Origin',(6.8,-0.25,-18.55));
#26185=CARTESIAN_POINT('',(-1.6,-0.5,-18.8));
#26186=CARTESIAN_POINT('Origin',(-1.6,-0.25,-16.8));
#26187=CARTESIAN_POINT('',(-3.6,-0.5,-16.8));
#26188=CARTESIAN_POINT('Origin',(-3.35,-0.25,8.4));
#26189=CARTESIAN_POINT('',(-3.6,-0.5,16.8));
#26190=CARTESIAN_POINT('Origin',(-1.6,-0.25,16.8));
#26191=CARTESIAN_POINT('',(-1.6,-0.5,18.8));
#26192=CARTESIAN_POINT('',(-1.6,-0.5,18.8));
#26193=CARTESIAN_POINT('Origin',(-1.6,-0.5,16.8));
#26194=CARTESIAN_POINT('Origin',(23.6,-0.25,18.55));
#26195=CARTESIAN_POINT('',(23.6,-0.5,18.8));
#26196=CARTESIAN_POINT('Origin',(32.,0.,16.8));
#26197=CARTESIAN_POINT('',(32.,-12.5,18.8));
#26198=CARTESIAN_POINT('',(32.,0.,18.8));
#26199=CARTESIAN_POINT('Origin',(32.,-12.5,16.8));
#26200=CARTESIAN_POINT('Origin',(-3.35,-8.,15.55));
#26201=CARTESIAN_POINT('',(-3.1,-19.,15.8));
#26202=CARTESIAN_POINT('',(-1.10000000000001,-17.,17.8));
#26203=CARTESIAN_POINT('',(-3.1,-13.,15.8));
#26204=CARTESIAN_POINT('',(-3.1,-8.,15.8));
#26205=CARTESIAN_POINT('',(-3.76666666666667,-12.3333333333333,15.1333333333333));
#26206=CARTESIAN_POINT('Origin',(15.2,-16.,15.8));
#26207=CARTESIAN_POINT('',(33.5,-19.,15.8));
#26208=CARTESIAN_POINT('',(-4.8,-19.,15.8));
#26209=CARTESIAN_POINT('',(33.5,-13.,15.8));
#26210=CARTESIAN_POINT('',(33.5,-8.,15.8));
#26211=CARTESIAN_POINT('',(35.2,-13.,15.8));
#26212=CARTESIAN_POINT('Origin',(33.75,-8.,15.55));
#26213=CARTESIAN_POINT('',(36.9666666666667,-9.53333333333332,12.3333333333333));
#26214=CARTESIAN_POINT('',(34.3,-19.8,15.));
#26215=CARTESIAN_POINT('Origin',(28.2,-69.75,-4.));
#26216=CARTESIAN_POINT('',(36.7,-70.,-4.));
#26217=CARTESIAN_POINT('',(37.2,-69.5,-4.));
#26218=CARTESIAN_POINT('',(28.2,-70.,-12.5));
#26219=CARTESIAN_POINT('Origin',(28.2,-70.,-4.));
#26220=CARTESIAN_POINT('',(28.2,-70.,-12.5));
#26221=CARTESIAN_POINT('Origin',(36.95,-69.75,-2.));
#26222=CARTESIAN_POINT('',(36.7,-70.,4.));
#26223=CARTESIAN_POINT('',(37.2,-69.5,4.));
#26224=CARTESIAN_POINT('',(36.7,-70.,-2.));
#26225=CARTESIAN_POINT('Origin',(28.2,-69.75,4.));
#26226=CARTESIAN_POINT('',(28.2,-70.,12.5));
#26227=CARTESIAN_POINT('',(28.2,-69.5,13.));
#26228=CARTESIAN_POINT('Origin',(28.2,-70.,4.));
#26229=CARTESIAN_POINT('Origin',(21.7,-69.75,12.75));
#26230=CARTESIAN_POINT('',(2.2,-70.,12.5));
#26231=CARTESIAN_POINT('',(2.2,-69.5,13.));
#26232=CARTESIAN_POINT('',(21.7,-70.,12.5));
#26233=CARTESIAN_POINT('',(21.7,-69.5,13.));
#26234=CARTESIAN_POINT('Origin',(2.2,-69.75,4.));
#26235=CARTESIAN_POINT('',(-6.3,-70.,4.));
#26236=CARTESIAN_POINT('',(-6.8,-69.5,4.));
#26237=CARTESIAN_POINT('Origin',(2.2,-70.,4.));
#26238=CARTESIAN_POINT('Origin',(-6.55,-69.75,2.));
#26239=CARTESIAN_POINT('',(-6.3,-70.,-4.));
#26240=CARTESIAN_POINT('',(-6.8,-69.5,-4.));
#26241=CARTESIAN_POINT('',(-6.3,-70.,2.));
#26242=CARTESIAN_POINT('Origin',(2.2,-69.75,-4.));
#26243=CARTESIAN_POINT('',(2.2,-70.,-12.5));
#26244=CARTESIAN_POINT('',(2.2,-69.5,-13.));
#26245=CARTESIAN_POINT('Origin',(2.2,-70.,-4.));
#26246=CARTESIAN_POINT('Origin',(8.7,-69.75,-12.75));
#26247=CARTESIAN_POINT('',(8.7,-70.,-12.5));
#26248=CARTESIAN_POINT('',(8.7,-69.5,-13.));
#26249=CARTESIAN_POINT('Origin',(28.2,-31.9,13.));
#26250=CARTESIAN_POINT('',(21.7,-31.9,13.));
#26251=CARTESIAN_POINT('Origin',(15.2,-70.,0.));
#26252=CARTESIAN_POINT('',(26.,-70.,9.8));
#26253=CARTESIAN_POINT('',(26.,-70.,-9.8));
#26254=CARTESIAN_POINT('',(26.,-70.,-4.65));
#26255=CARTESIAN_POINT('',(34.4,-70.,9.8));
#26256=CARTESIAN_POINT('',(20.85,-70.,9.8));
#26257=CARTESIAN_POINT('',(34.4,-70.,-9.8));
#26258=CARTESIAN_POINT('',(34.4,-70.,4.65));
#26259=CARTESIAN_POINT('',(24.55,-70.,-9.8));
#26260=CARTESIAN_POINT('',(6.,-70.,9.8));
#26261=CARTESIAN_POINT('',(6.,-70.,-9.8));
#26262=CARTESIAN_POINT('',(6.,-70.,-4.65));
#26263=CARTESIAN_POINT('',(14.4,-70.,9.8));
#26264=CARTESIAN_POINT('',(10.85,-70.,9.8));
#26265=CARTESIAN_POINT('',(14.4,-70.,-9.8));
#26266=CARTESIAN_POINT('',(14.4,-70.,4.65));
#26267=CARTESIAN_POINT('',(14.55,-70.,-9.8));
#26268=CARTESIAN_POINT('',(16.,-70.,9.8));
#26269=CARTESIAN_POINT('',(16.,-70.,-9.8));
#26270=CARTESIAN_POINT('',(16.,-70.,-4.65));
#26271=CARTESIAN_POINT('',(24.4,-70.,9.8));
#26272=CARTESIAN_POINT('',(15.85,-70.,9.8));
#26273=CARTESIAN_POINT('',(24.4,-70.,-9.8));
#26274=CARTESIAN_POINT('',(24.4,-70.,4.65));
#26275=CARTESIAN_POINT('',(19.55,-70.,-9.8));
#26276=CARTESIAN_POINT('',(-4.,-70.,9.8));
#26277=CARTESIAN_POINT('',(-4.,-70.,-9.8));
#26278=CARTESIAN_POINT('',(-4.,-70.,-4.65));
#26279=CARTESIAN_POINT('',(4.4,-70.,9.8));
#26280=CARTESIAN_POINT('',(5.85,-70.,9.8));
#26281=CARTESIAN_POINT('',(4.4,-70.,-9.8));
#26282=CARTESIAN_POINT('',(4.4,-70.,4.65));
#26283=CARTESIAN_POINT('',(9.55,-70.,-9.8));
#26284=CARTESIAN_POINT('Origin',(-3.35,-12.75,17.8));
#26285=CARTESIAN_POINT('',(-3.1,-13.,16.8));
#26286=CARTESIAN_POINT('',(-3.1,-13.,17.8));
#26287=CARTESIAN_POINT('',(-3.1,-13.,16.8));
#26288=CARTESIAN_POINT('Origin',(-1.6,-12.75,16.8));
#26289=CARTESIAN_POINT('',(-1.6,-13.,18.3));
#26290=CARTESIAN_POINT('',(-1.6,-12.5,18.8));
#26291=CARTESIAN_POINT('',(-1.6,-13.,18.3));
#26292=CARTESIAN_POINT('Origin',(-1.6,-12.5,16.8));
#26293=CARTESIAN_POINT('Origin',(-1.6,-13.,16.8));
#26294=CARTESIAN_POINT('Origin',(13.6,-12.75,18.55));
#26295=CARTESIAN_POINT('',(32.,-13.,18.3));
#26296=CARTESIAN_POINT('',(32.,-13.,18.3));
#26297=CARTESIAN_POINT('',(13.6,-12.5,18.8));
#26298=CARTESIAN_POINT('',(13.6,-13.,18.3));
#26299=CARTESIAN_POINT('Origin',(32.,-12.75,16.8));
#26300=CARTESIAN_POINT('',(33.5,-13.,16.8));
#26301=CARTESIAN_POINT('',(33.5,-13.,16.8));
#26302=CARTESIAN_POINT('Origin',(32.,-13.,16.8));
#26303=CARTESIAN_POINT('Origin',(33.75,-12.75,1.));
#26304=CARTESIAN_POINT('',(33.5,-13.,1.));
#26305=CARTESIAN_POINT('Origin',(-4.8,-13.,18.8));
#26306=CARTESIAN_POINT('Origin',(33.75,-19.25,1.));
#26307=CARTESIAN_POINT('',(33.5,-19.,16.8));
#26308=CARTESIAN_POINT('',(33.5,-19.,1.));
#26309=CARTESIAN_POINT('',(33.5,-19.,16.8));
#26310=CARTESIAN_POINT('Origin',(32.,-19.25,16.8));
#26311=CARTESIAN_POINT('',(32.,-19.,18.3));
#26312=CARTESIAN_POINT('',(32.,-19.,18.3));
#26313=CARTESIAN_POINT('Origin',(32.,-19.,16.8));
#26314=CARTESIAN_POINT('Origin',(33.6,-19.25,18.55));
#26315=CARTESIAN_POINT('',(-1.6,-19.,18.3));
#26316=CARTESIAN_POINT('',(-1.6,-19.,18.3));
#26317=CARTESIAN_POINT('',(33.6,-19.,18.3));
#26318=CARTESIAN_POINT('Origin',(-1.6,-19.25,16.8));
#26319=CARTESIAN_POINT('',(-3.1,-19.,16.8));
#26320=CARTESIAN_POINT('',(-3.1,-19.,16.8));
#26321=CARTESIAN_POINT('Origin',(-1.6,-19.,16.8));
#26322=CARTESIAN_POINT('Origin',(-3.35,-19.25,17.8));
#26323=CARTESIAN_POINT('',(-3.1,-19.,17.8));
#26324=CARTESIAN_POINT('Origin',(35.2,-19.,18.8));
#26325=CARTESIAN_POINT('Origin',(34.15,-69.75,4.65));
#26326=CARTESIAN_POINT('',(33.9,-69.5,9.3));
#26327=CARTESIAN_POINT('',(34.4,-70.,9.8));
#26328=CARTESIAN_POINT('',(33.9,-69.5,-9.3));
#26329=CARTESIAN_POINT('',(33.9,-69.5,4.65));
#26330=CARTESIAN_POINT('',(34.4,-70.,-9.8));
#26331=CARTESIAN_POINT('Origin',(26.25,-69.75,-4.65));
#26332=CARTESIAN_POINT('',(26.5,-69.5,-9.3));
#26333=CARTESIAN_POINT('',(26.,-70.,-9.8));
#26334=CARTESIAN_POINT('',(26.5,-69.5,9.3));
#26335=CARTESIAN_POINT('',(26.5,-69.5,-4.65));
#26336=CARTESIAN_POINT('',(26.5,-69.5,9.3));
#26337=CARTESIAN_POINT('Origin',(24.55,-69.75,-9.55));
#26338=CARTESIAN_POINT('',(24.55,-69.5,-9.3));
#26339=CARTESIAN_POINT('Origin',(20.85,-69.75,9.55));
#26340=CARTESIAN_POINT('',(20.85,-69.5,9.3));
#26341=CARTESIAN_POINT('Origin',(26.5,-70.,9.3));
#26342=CARTESIAN_POINT('',(26.5,-52.,9.3));
#26343=CARTESIAN_POINT('',(26.5,-70.,9.3));
#26344=CARTESIAN_POINT('',(33.9,-52.,9.3));
#26345=CARTESIAN_POINT('',(33.9,-52.,9.3));
#26346=CARTESIAN_POINT('',(33.9,-70.,9.3));
#26347=CARTESIAN_POINT('Origin',(26.5,-70.,-9.3));
#26348=CARTESIAN_POINT('',(26.5,-52.,-9.3));
#26349=CARTESIAN_POINT('',(26.5,-70.,-9.3));
#26350=CARTESIAN_POINT('',(26.5,-52.,9.3));
#26351=CARTESIAN_POINT('',(26.5,-61.,1.525));
#26352=CARTESIAN_POINT('Origin',(26.5,-61.,0.));
#26353=CARTESIAN_POINT('Origin',(4.15,-69.75,4.65));
#26354=CARTESIAN_POINT('',(3.9,-69.5,9.3));
#26355=CARTESIAN_POINT('',(4.4,-70.,9.8));
#26356=CARTESIAN_POINT('',(3.9,-69.5,-9.3));
#26357=CARTESIAN_POINT('',(3.9,-69.5,4.65));
#26358=CARTESIAN_POINT('',(4.4,-70.,-9.8));
#26359=CARTESIAN_POINT('Origin',(-3.75,-69.75,-4.65));
#26360=CARTESIAN_POINT('',(-3.5,-69.5,-9.3));
#26361=CARTESIAN_POINT('',(-4.,-70.,-9.8));
#26362=CARTESIAN_POINT('',(-3.5,-69.5,9.3));
#26363=CARTESIAN_POINT('',(-3.5,-69.5,-4.65));
#26364=CARTESIAN_POINT('',(-3.5,-69.5,9.3));
#26365=CARTESIAN_POINT('Origin',(9.55,-69.75,-9.55));
#26366=CARTESIAN_POINT('',(9.55,-69.5,-9.3));
#26367=CARTESIAN_POINT('Origin',(5.85,-69.75,9.55));
#26368=CARTESIAN_POINT('',(5.85,-69.5,9.3));
#26369=CARTESIAN_POINT('Origin',(-3.5,-70.,9.3));
#26370=CARTESIAN_POINT('',(-3.5,-52.,9.3));
#26371=CARTESIAN_POINT('',(-3.5,-70.,9.3));
#26372=CARTESIAN_POINT('',(3.9,-52.,9.3));
#26373=CARTESIAN_POINT('',(3.9,-52.,9.3));
#26374=CARTESIAN_POINT('',(3.9,-70.,9.3));
#26375=CARTESIAN_POINT('Origin',(-3.5,-70.,-9.3));
#26376=CARTESIAN_POINT('',(-3.5,-52.,-9.3));
#26377=CARTESIAN_POINT('',(-3.5,-70.,-9.3));
#26378=CARTESIAN_POINT('',(-3.5,-52.,9.3));
#26379=CARTESIAN_POINT('',(-3.5,-61.,1.525));
#26380=CARTESIAN_POINT('Origin',(-3.5,-61.,0.));
#26381=CARTESIAN_POINT('Origin',(14.15,-69.75,4.65));
#26382=CARTESIAN_POINT('',(13.9,-69.5,9.3));
#26383=CARTESIAN_POINT('',(14.4,-70.,9.8));
#26384=CARTESIAN_POINT('',(13.9,-69.5,-9.3));
#26385=CARTESIAN_POINT('',(13.9,-69.5,4.65));
#26386=CARTESIAN_POINT('',(14.4,-70.,-9.8));
#26387=CARTESIAN_POINT('Origin',(6.25,-69.75,-4.65));
#26388=CARTESIAN_POINT('',(6.5,-69.5,-9.3));
#26389=CARTESIAN_POINT('',(6.,-70.,-9.8));
#26390=CARTESIAN_POINT('',(6.5,-69.5,9.3));
#26391=CARTESIAN_POINT('',(6.5,-69.5,-4.65));
#26392=CARTESIAN_POINT('',(6.5,-69.5,9.3));
#26393=CARTESIAN_POINT('Origin',(14.55,-69.75,-9.55));
#26394=CARTESIAN_POINT('',(14.55,-69.5,-9.3));
#26395=CARTESIAN_POINT('Origin',(10.85,-69.75,9.55));
#26396=CARTESIAN_POINT('',(10.85,-69.5,9.3));
#26397=CARTESIAN_POINT('Origin',(6.5,-70.,9.3));
#26398=CARTESIAN_POINT('',(6.5,-52.,9.3));
#26399=CARTESIAN_POINT('',(6.5,-70.,9.3));
#26400=CARTESIAN_POINT('',(13.9,-52.,9.3));
#26401=CARTESIAN_POINT('',(13.9,-52.,9.3));
#26402=CARTESIAN_POINT('',(13.9,-70.,9.3));
#26403=CARTESIAN_POINT('Origin',(6.5,-70.,-9.3));
#26404=CARTESIAN_POINT('',(6.5,-52.,-9.3));
#26405=CARTESIAN_POINT('',(6.5,-70.,-9.3));
#26406=CARTESIAN_POINT('',(6.5,-52.,9.3));
#26407=CARTESIAN_POINT('',(6.5,-61.,1.525));
#26408=CARTESIAN_POINT('Origin',(6.5,-61.,0.));
#26409=CARTESIAN_POINT('Origin',(24.15,-69.75,4.65));
#26410=CARTESIAN_POINT('',(23.9,-69.5,9.3));
#26411=CARTESIAN_POINT('',(24.4,-70.,9.8));
#26412=CARTESIAN_POINT('',(23.9,-69.5,-9.3));
#26413=CARTESIAN_POINT('',(23.9,-69.5,4.65));
#26414=CARTESIAN_POINT('',(24.4,-70.,-9.8));
#26415=CARTESIAN_POINT('Origin',(16.25,-69.75,-4.65));
#26416=CARTESIAN_POINT('',(16.5,-69.5,-9.3));
#26417=CARTESIAN_POINT('',(16.,-70.,-9.8));
#26418=CARTESIAN_POINT('',(16.5,-69.5,9.3));
#26419=CARTESIAN_POINT('',(16.5,-69.5,-4.65));
#26420=CARTESIAN_POINT('',(16.5,-69.5,9.3));
#26421=CARTESIAN_POINT('Origin',(19.55,-69.75,-9.55));
#26422=CARTESIAN_POINT('',(19.55,-69.5,-9.3));
#26423=CARTESIAN_POINT('Origin',(15.85,-69.75,9.55));
#26424=CARTESIAN_POINT('',(15.85,-69.5,9.3));
#26425=CARTESIAN_POINT('Origin',(16.5,-70.,9.3));
#26426=CARTESIAN_POINT('',(16.5,-52.,9.3));
#26427=CARTESIAN_POINT('',(16.5,-70.,9.3));
#26428=CARTESIAN_POINT('',(23.9,-52.,9.3));
#26429=CARTESIAN_POINT('',(23.9,-52.,9.3));
#26430=CARTESIAN_POINT('',(23.9,-70.,9.3));
#26431=CARTESIAN_POINT('Origin',(16.5,-70.,-9.3));
#26432=CARTESIAN_POINT('',(16.5,-52.,-9.3));
#26433=CARTESIAN_POINT('',(16.5,-70.,-9.3));
#26434=CARTESIAN_POINT('',(16.5,-52.,9.3));
#26435=CARTESIAN_POINT('',(16.5,-61.,1.525));
#26436=CARTESIAN_POINT('Origin',(16.5,-61.,0.));
#26437=CARTESIAN_POINT('Origin',(37.3,-61.,0.));
#26438=CARTESIAN_POINT('',(33.9,-61.,1.525));
#26439=CARTESIAN_POINT('',(37.3,-61.,1.525));
#26440=CARTESIAN_POINT('Origin',(33.9,-61.,0.));
#26441=CARTESIAN_POINT('Origin',(37.3,-61.,0.));
#26442=CARTESIAN_POINT('',(3.9,-61.,1.525));
#26443=CARTESIAN_POINT('',(37.3,-61.,1.525));
#26444=CARTESIAN_POINT('Origin',(3.9,-61.,0.));
#26445=CARTESIAN_POINT('Origin',(37.3,-61.,0.));
#26446=CARTESIAN_POINT('',(13.9,-61.,1.525));
#26447=CARTESIAN_POINT('',(37.3,-61.,1.525));
#26448=CARTESIAN_POINT('Origin',(13.9,-61.,0.));
#26449=CARTESIAN_POINT('Origin',(37.3,-61.,0.));
#26450=CARTESIAN_POINT('',(23.9,-61.,1.525));
#26451=CARTESIAN_POINT('',(37.3,-61.,1.525));
#26452=CARTESIAN_POINT('Origin',(23.9,-61.,0.));
#26453=CARTESIAN_POINT('Origin',(37.3,-61.,0.));
#26454=CARTESIAN_POINT('',(37.3,-61.,1.525));
#26455=CARTESIAN_POINT('Origin',(23.9,-70.,-9.3));
#26456=CARTESIAN_POINT('',(23.9,-52.,-9.3));
#26457=CARTESIAN_POINT('',(23.9,-70.,-9.3));
#26458=CARTESIAN_POINT('',(16.5,-52.,-9.3));
#26459=CARTESIAN_POINT('Origin',(23.9,-70.,9.3));
#26460=CARTESIAN_POINT('',(23.9,-52.,-9.3));
#26461=CARTESIAN_POINT('Origin',(20.2,-52.,0.));
#26462=CARTESIAN_POINT('Origin',(13.9,-70.,-9.3));
#26463=CARTESIAN_POINT('',(13.9,-52.,-9.3));
#26464=CARTESIAN_POINT('',(13.9,-70.,-9.3));
#26465=CARTESIAN_POINT('',(6.5,-52.,-9.3));
#26466=CARTESIAN_POINT('Origin',(13.9,-70.,9.3));
#26467=CARTESIAN_POINT('',(13.9,-52.,-9.3));
#26468=CARTESIAN_POINT('Origin',(10.2,-52.,0.));
#26469=CARTESIAN_POINT('Origin',(3.9,-70.,-9.3));
#26470=CARTESIAN_POINT('',(3.9,-52.,-9.3));
#26471=CARTESIAN_POINT('',(3.9,-70.,-9.3));
#26472=CARTESIAN_POINT('',(-3.5,-52.,-9.3));
#26473=CARTESIAN_POINT('Origin',(3.9,-70.,9.3));
#26474=CARTESIAN_POINT('',(3.9,-52.,-9.3));
#26475=CARTESIAN_POINT('Origin',(0.199999999999999,-52.,0.));
#26476=CARTESIAN_POINT('Origin',(33.9,-70.,-9.3));
#26477=CARTESIAN_POINT('',(33.9,-52.,-9.3));
#26478=CARTESIAN_POINT('',(33.9,-70.,-9.3));
#26479=CARTESIAN_POINT('',(26.5,-52.,-9.3));
#26480=CARTESIAN_POINT('Origin',(33.9,-70.,9.3));
#26481=CARTESIAN_POINT('',(33.9,-52.,-9.3));
#26482=CARTESIAN_POINT('Origin',(30.2,-52.,0.));
#26483=CARTESIAN_POINT('Origin',(32.,0.,18.8));
#26484=CARTESIAN_POINT('',(-1.6,0.,18.8));
#26485=CARTESIAN_POINT('Origin',(-1.6,0.,16.8));
#26486=CARTESIAN_POINT('Origin',(15.2,-32.5,0.));
#26487=CARTESIAN_POINT('Origin',(15.2,-31.9,0.));
#26488=CARTESIAN_POINT('Origin',(15.2,-31.9,0.));
#26489=CARTESIAN_POINT('Origin',(2.2,-31.9,-13.));
#26490=CARTESIAN_POINT('',(8.7,-31.9,-13.));
#26491=CARTESIAN_POINT('Origin',(15.2,-31.9,-2.22044604925031E-15));
#26492=CARTESIAN_POINT('Origin',(15.2,-31.9,-2.22044604925031E-15));
#32286=UNCERTAINTY_MEASURE_WITH_UNIT(LENGTH_MEASURE(0.01),#32310,
'DISTANCE_ACCURACY_VALUE',
'Maximum model space distance between geometric entities at asserted c
onnectivities');
#32293=UNCERTAINTY_MEASURE_WITH_UNIT(LENGTH_MEASURE(0.01),#32310,
'DISTANCE_ACCURACY_VALUE',
'Maximum model space distance between geometric entities at asserted c
onnectivities');
#32302=(
GEOMETRIC_REPRESENTATION_CONTEXT(3)
GLOBAL_UNCERTAINTY_ASSIGNED_CONTEXT((#32286))
GLOBAL_UNIT_ASSIGNED_CONTEXT((#32310,#32312,#32313))
REPRESENTATION_CONTEXT('','3D')
);
#32309=(
GEOMETRIC_REPRESENTATION_CONTEXT(3)
GLOBAL_UNCERTAINTY_ASSIGNED_CONTEXT((#32293))
GLOBAL_UNIT_ASSIGNED_CONTEXT((#32310,#32312,#32313))
REPRESENTATION_CONTEXT('','3D')
);
#32310=(
LENGTH_UNIT()
NAMED_UNIT(*)
SI_UNIT(.MILLI.,.METRE.)
);
#32312=(
NAMED_UNIT(*)
PLANE_ANGLE_UNIT()
SI_UNIT($,.RADIAN.)
);
#32313=(
NAMED_UNIT(*)
SI_UNIT($,.STERADIAN.)
SOLID_ANGLE_UNIT()
);
#32322=SHAPE_DEFINITION_REPRESENTATION(#32337,#32369);
#32337=PRODUCT_DEFINITION_SHAPE('',$,#32385);
#32369=SHAPE_REPRESENTATION('',(#14432),#32302);
#32376=PRODUCT_DEFINITION_CONTEXT('part definition',#32423,'design');
#32385=PRODUCT_DEFINITION('2026-10-25-00-35-18-111',
'08_Combination_Barrel_Lock_Body',#32400,#32376);
#32400=PRODUCT_DEFINITION_FORMATION('',$,#32433);
#32423=APPLICATION_CONTEXT(
'Core Data for Automotive Mechanical Design Process');
#32424=PRODUCT_CONTEXT('part definition',#32423,'mechanical');
#32433=PRODUCT('2026-10-25-00-35-18-111',
'08_Combination_Barrel_Lock_Body',$,(#32424));
#32475=COLOUR_RGB('Dark Blue',0.08,0.2,0.34);
#32476=FILL_AREA_STYLE_COLOUR('',#32475);
#32477=FILL_AREA_STYLE('',(#32476));
#32478=SURFACE_STYLE_FILL_AREA(#32477);
#32479=SURFACE_SIDE_STYLE('',(#32478));
#32480=SURFACE_STYLE_USAGE(.BOTH.,#32479);
#32481=PRESENTATION_STYLE_ASSIGNMENT((#32480));
ENDSEC;
END-ISO-10303-21;
